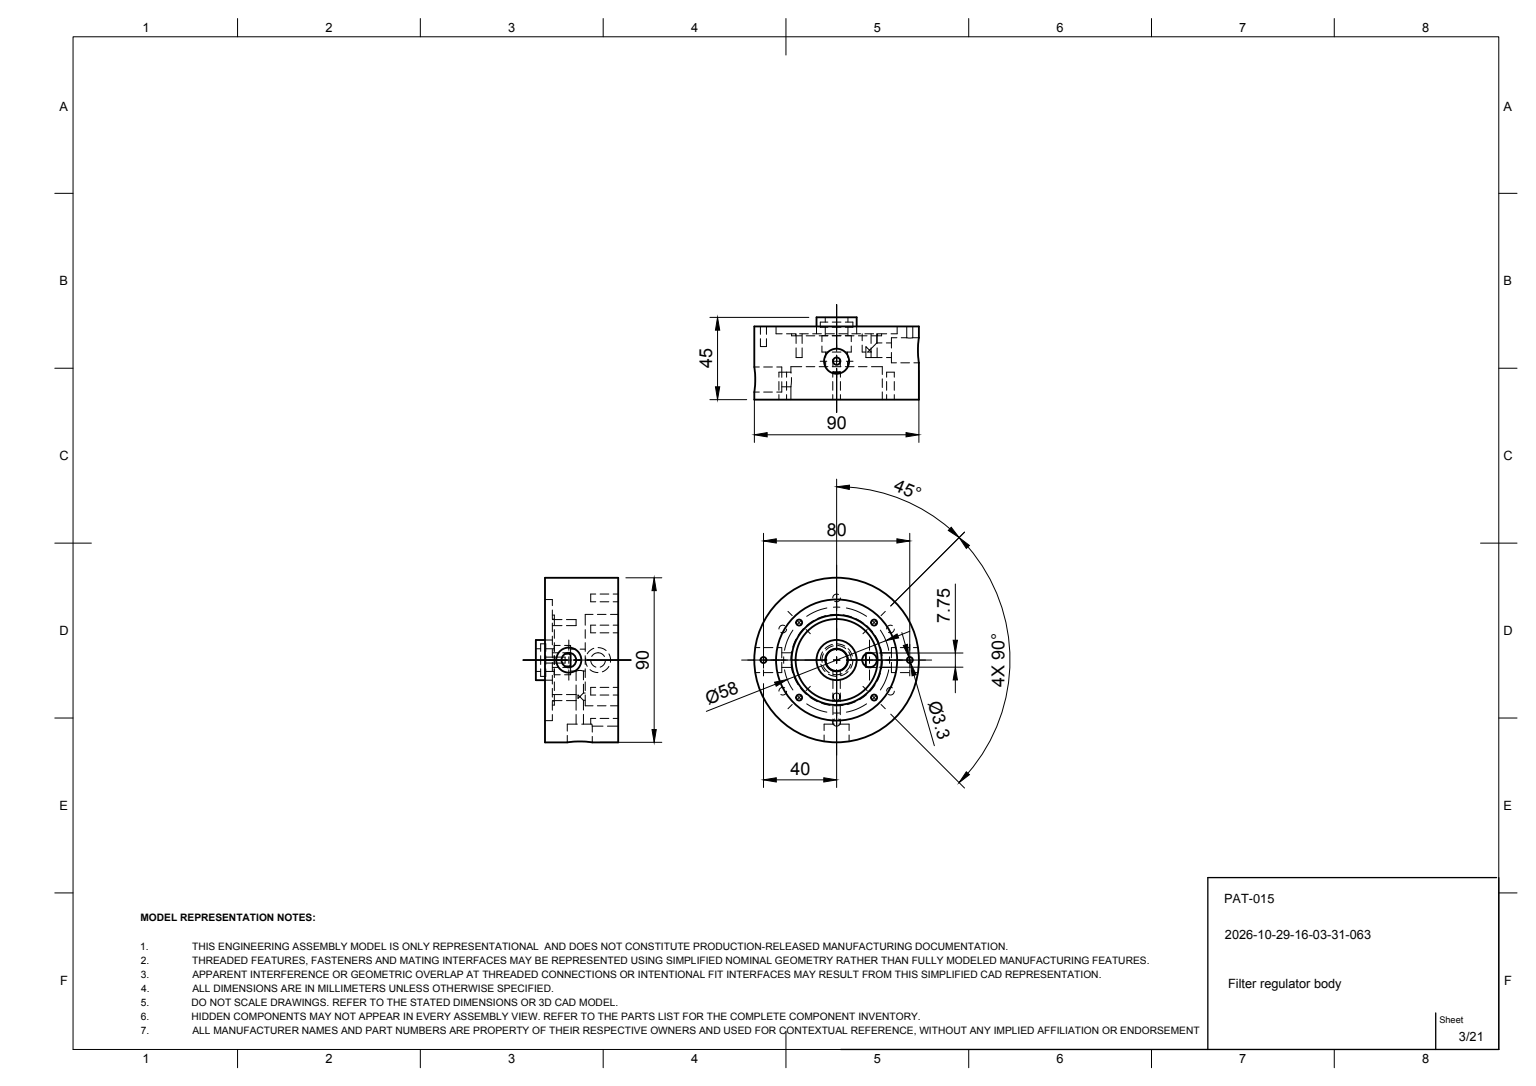
ISO-10303-21;
HEADER;
/* Generated by software containing ST-Developer
 * from STEP Tools, Inc. (www.steptools.com) 
 */

FILE_DESCRIPTION(
/* description */ ('PAT-015'),
/* implementation_level */ '2;1');

FILE_NAME(
/* name */ 'Filter regulator body.step',
/* time_stamp */ '2026-10-29T16:03:43-07:00',
/* author */ (''),
/* organization */ (''),
/* preprocessor_version */ 'ST-DEVELOPER v20.2',
/* originating_system */ 'Autodesk Translation Framework v15.17.0.0',
/* authorisation */ '');

FILE_SCHEMA (('AUTOMOTIVE_DESIGN { 1 0 10303 214 3 1 1 }'));
ENDSEC;

DATA;
#10=MECHANICAL_DESIGN_GEOMETRIC_PRESENTATION_REPRESENTATION('',(#230),#10266);
#184=SHAPE_REPRESENTATION_RELATIONSHIP('SRR','None',#10355,#207);
#207=ADVANCED_BREP_SHAPE_REPRESENTATION('',(#255),#10243);
#230=STYLED_ITEM('',(#10526),#255);
#255=MANIFOLD_SOLID_BREP('Body1',#4689);
#278=ELLIPSE('',#5037,0.282842712474619,0.2);
#279=ELLIPSE('',#5038,0.282842712474619,0.2);
#280=ELLIPSE('',#5040,0.282842712474619,0.2);
#281=ELLIPSE('',#5041,0.282842712474619,0.2);
#282=ELLIPSE('',#5043,0.282842712474619,0.2);
#283=ELLIPSE('',#5045,0.282842712474619,0.2);
#284=ELLIPSE('',#5060,0.565685424949238,0.4);
#285=ELLIPSE('',#5061,0.565685424949238,0.4);
#286=ELLIPSE('',#5063,0.565685424949238,0.4);
#287=ELLIPSE('',#5064,0.565685424949238,0.4);
#288=ELLIPSE('',#5067,0.565685424949238,0.4);
#289=ELLIPSE('',#5068,0.565685424949238,0.4);
#290=ELLIPSE('',#5069,0.565685424949238,0.4);
#291=ELLIPSE('',#5070,0.565685424949238,0.4);
#292=FACE_BOUND('',#868,.T.);
#293=FACE_BOUND('',#870,.T.);
#294=FACE_BOUND('',#871,.T.);
#295=FACE_BOUND('',#872,.T.);
#296=FACE_BOUND('',#873,.T.);
#297=FACE_BOUND('',#874,.T.);
#298=FACE_BOUND('',#888,.T.);
#299=FACE_BOUND('',#899,.T.);
#300=FACE_BOUND('',#909,.T.);
#301=FACE_BOUND('',#911,.T.);
#302=FACE_BOUND('',#914,.T.);
#303=FACE_BOUND('',#916,.T.);
#304=FACE_BOUND('',#921,.T.);
#305=FACE_BOUND('',#923,.T.);
#306=FACE_BOUND('',#925,.T.);
#307=FACE_BOUND('',#928,.T.);
#308=FACE_BOUND('',#930,.T.);
#309=FACE_BOUND('',#932,.T.);
#310=FACE_BOUND('',#933,.T.);
#311=FACE_BOUND('',#936,.T.);
#312=FACE_BOUND('',#937,.T.);
#313=FACE_BOUND('',#939,.T.);
#314=FACE_BOUND('',#940,.T.);
#315=FACE_BOUND('',#942,.T.);
#316=FACE_BOUND('',#943,.T.);
#317=FACE_BOUND('',#944,.T.);
#318=FACE_BOUND('',#945,.T.);
#319=FACE_BOUND('',#946,.T.);
#320=FACE_BOUND('',#947,.T.);
#321=FACE_BOUND('',#948,.T.);
#322=FACE_BOUND('',#950,.T.);
#323=FACE_BOUND('',#951,.T.);
#324=FACE_BOUND('',#952,.T.);
#420=PLANE('',#4977);
#421=PLANE('',#4981);
#422=PLANE('',#4985);
#423=PLANE('',#4989);
#424=PLANE('',#4993);
#425=PLANE('',#5000);
#426=PLANE('',#5001);
#427=PLANE('',#5003);
#428=PLANE('',#5011);
#429=PLANE('',#5015);
#430=PLANE('',#5019);
#431=PLANE('',#5023);
#432=PLANE('',#5027);
#433=PLANE('',#5028);
#434=PLANE('',#5032);
#435=PLANE('',#5034);
#436=PLANE('',#5052);
#437=PLANE('',#5053);
#438=PLANE('',#5055);
#439=PLANE('',#5057);
#440=PLANE('',#5071);
#441=PLANE('',#5078);
#442=PLANE('',#5082);
#443=PLANE('',#5084);
#444=PLANE('',#5093);
#445=PLANE('',#5095);
#446=PLANE('',#5101);
#447=PLANE('',#5105);
#448=PLANE('',#5108);
#449=PLANE('',#5112);
#450=PLANE('',#5113);
#571=FACE_OUTER_BOUND('',#854,.T.);
#572=FACE_OUTER_BOUND('',#855,.T.);
#573=FACE_OUTER_BOUND('',#856,.T.);
#574=FACE_OUTER_BOUND('',#857,.T.);
#575=FACE_OUTER_BOUND('',#858,.T.);
#576=FACE_OUTER_BOUND('',#859,.T.);
#577=FACE_OUTER_BOUND('',#860,.T.);
#578=FACE_OUTER_BOUND('',#861,.T.);
#579=FACE_OUTER_BOUND('',#862,.T.);
#580=FACE_OUTER_BOUND('',#863,.T.);
#581=FACE_OUTER_BOUND('',#864,.T.);
#582=FACE_OUTER_BOUND('',#865,.T.);
#583=FACE_OUTER_BOUND('',#866,.T.);
#584=FACE_OUTER_BOUND('',#867,.T.);
#585=FACE_OUTER_BOUND('',#869,.T.);
#586=FACE_OUTER_BOUND('',#875,.T.);
#587=FACE_OUTER_BOUND('',#876,.T.);
#588=FACE_OUTER_BOUND('',#877,.T.);
#589=FACE_OUTER_BOUND('',#878,.T.);
#590=FACE_OUTER_BOUND('',#879,.T.);
#591=FACE_OUTER_BOUND('',#880,.T.);
#592=FACE_OUTER_BOUND('',#881,.T.);
#593=FACE_OUTER_BOUND('',#882,.T.);
#594=FACE_OUTER_BOUND('',#883,.T.);
#595=FACE_OUTER_BOUND('',#884,.T.);
#596=FACE_OUTER_BOUND('',#885,.T.);
#597=FACE_OUTER_BOUND('',#886,.T.);
#598=FACE_OUTER_BOUND('',#887,.T.);
#599=FACE_OUTER_BOUND('',#889,.T.);
#600=FACE_OUTER_BOUND('',#890,.T.);
#601=FACE_OUTER_BOUND('',#891,.T.);
#602=FACE_OUTER_BOUND('',#892,.T.);
#603=FACE_OUTER_BOUND('',#893,.T.);
#604=FACE_OUTER_BOUND('',#894,.T.);
#605=FACE_OUTER_BOUND('',#895,.T.);
#606=FACE_OUTER_BOUND('',#896,.T.);
#607=FACE_OUTER_BOUND('',#897,.T.);
#608=FACE_OUTER_BOUND('',#898,.T.);
#609=FACE_OUTER_BOUND('',#900,.T.);
#610=FACE_OUTER_BOUND('',#901,.T.);
#611=FACE_OUTER_BOUND('',#902,.T.);
#612=FACE_OUTER_BOUND('',#903,.T.);
#613=FACE_OUTER_BOUND('',#904,.T.);
#614=FACE_OUTER_BOUND('',#905,.T.);
#615=FACE_OUTER_BOUND('',#906,.T.);
#616=FACE_OUTER_BOUND('',#907,.T.);
#617=FACE_OUTER_BOUND('',#908,.T.);
#618=FACE_OUTER_BOUND('',#910,.T.);
#619=FACE_OUTER_BOUND('',#912,.T.);
#620=FACE_OUTER_BOUND('',#913,.T.);
#621=FACE_OUTER_BOUND('',#915,.T.);
#622=FACE_OUTER_BOUND('',#917,.T.);
#623=FACE_OUTER_BOUND('',#918,.T.);
#624=FACE_OUTER_BOUND('',#919,.T.);
#625=FACE_OUTER_BOUND('',#920,.T.);
#626=FACE_OUTER_BOUND('',#922,.T.);
#627=FACE_OUTER_BOUND('',#924,.T.);
#628=FACE_OUTER_BOUND('',#926,.T.);
#629=FACE_OUTER_BOUND('',#927,.T.);
#630=FACE_OUTER_BOUND('',#929,.T.);
#631=FACE_OUTER_BOUND('',#931,.T.);
#632=FACE_OUTER_BOUND('',#934,.T.);
#633=FACE_OUTER_BOUND('',#935,.T.);
#634=FACE_OUTER_BOUND('',#938,.T.);
#635=FACE_OUTER_BOUND('',#941,.T.);
#636=FACE_OUTER_BOUND('',#949,.T.);
#854=EDGE_LOOP('',(#3101,#3102,#3103,#3104,#3105));
#855=EDGE_LOOP('',(#3106,#3107,#3108,#3109));
#856=EDGE_LOOP('',(#3110));
#857=EDGE_LOOP('',(#3111,#3112,#3113,#3114));
#858=EDGE_LOOP('',(#3115));
#859=EDGE_LOOP('',(#3116,#3117,#3118,#3119));
#860=EDGE_LOOP('',(#3120));
#861=EDGE_LOOP('',(#3121,#3122,#3123,#3124));
#862=EDGE_LOOP('',(#3125));
#863=EDGE_LOOP('',(#3126,#3127,#3128,#3129));
#864=EDGE_LOOP('',(#3130));
#865=EDGE_LOOP('',(#3131,#3132,#3133,#3134));
#866=EDGE_LOOP('',(#3135,#3136,#3137,#3138));
#867=EDGE_LOOP('',(#3139));
#868=EDGE_LOOP('',(#3140));
#869=EDGE_LOOP('',(#3141));
#870=EDGE_LOOP('',(#3142));
#871=EDGE_LOOP('',(#3143));
#872=EDGE_LOOP('',(#3144));
#873=EDGE_LOOP('',(#3145));
#874=EDGE_LOOP('',(#3146));
#875=EDGE_LOOP('',(#3147,#3148,#3149));
#876=EDGE_LOOP('',(#3150,#3151,#3152,#3153,#3154,#3155,#3156,#3157));
#877=EDGE_LOOP('',(#3158,#3159,#3160,#3161));
#878=EDGE_LOOP('',(#3162));
#879=EDGE_LOOP('',(#3163,#3164,#3165,#3166));
#880=EDGE_LOOP('',(#3167));
#881=EDGE_LOOP('',(#3168,#3169,#3170,#3171));
#882=EDGE_LOOP('',(#3172));
#883=EDGE_LOOP('',(#3173,#3174,#3175,#3176));
#884=EDGE_LOOP('',(#3177));
#885=EDGE_LOOP('',(#3178,#3179,#3180,#3181));
#886=EDGE_LOOP('',(#3182));
#887=EDGE_LOOP('',(#3183,#3184,#3185,#3186,#3187));
#888=EDGE_LOOP('',(#3188));
#889=EDGE_LOOP('',(#3189,#3190));
#890=EDGE_LOOP('',(#3191,#3192));
#891=EDGE_LOOP('',(#3193,#3194,#3195));
#892=EDGE_LOOP('',(#3196,#3197,#3198));
#893=EDGE_LOOP('',(#3199,#3200,#3201,#3202,#3203));
#894=EDGE_LOOP('',(#3204,#3205,#3206,#3207,#3208,#3209,#3210,#3211,#3212,
#3213,#3214,#3215,#3216,#3217));
#895=EDGE_LOOP('',(#3218,#3219,#3220,#3221,#3222,#3223));
#896=EDGE_LOOP('',(#3224,#3225,#3226,#3227,#3228));
#897=EDGE_LOOP('',(#3229,#3230,#3231,#3232,#3233));
#898=EDGE_LOOP('',(#3234));
#899=EDGE_LOOP('',(#3235));
#900=EDGE_LOOP('',(#3236,#3237));
#901=EDGE_LOOP('',(#3238,#3239));
#902=EDGE_LOOP('',(#3240,#3241));
#903=EDGE_LOOP('',(#3242,#3243,#3244));
#904=EDGE_LOOP('',(#3245,#3246,#3247));
#905=EDGE_LOOP('',(#3248,#3249,#3250,#3251,#3252,#3253,#3254,#3255,#3256,
#3257));
#906=EDGE_LOOP('',(#3258,#3259,#3260,#3261,#3262));
#907=EDGE_LOOP('',(#3263,#3264,#3265,#3266,#3267,#3268,#3269,#3270,#3271,
#3272,#3273,#3274,#3275,#3276,#3277));
#908=EDGE_LOOP('',(#3278,#3279,#3280,#3281,#3282,#3283));
#909=EDGE_LOOP('',(#3284,#3285));
#910=EDGE_LOOP('',(#3286));
#911=EDGE_LOOP('',(#3287));
#912=EDGE_LOOP('',(#3288,#3289,#3290,#3291));
#913=EDGE_LOOP('',(#3292));
#914=EDGE_LOOP('',(#3293));
#915=EDGE_LOOP('',(#3294));
#916=EDGE_LOOP('',(#3295));
#917=EDGE_LOOP('',(#3296,#3297,#3298,#3299));
#918=EDGE_LOOP('',(#3300,#3301,#3302,#3303));
#919=EDGE_LOOP('',(#3304,#3305,#3306,#3307));
#920=EDGE_LOOP('',(#3308));
#921=EDGE_LOOP('',(#3309));
#922=EDGE_LOOP('',(#3310));
#923=EDGE_LOOP('',(#3311));
#924=EDGE_LOOP('',(#3312,#3313,#3314,#3315));
#925=EDGE_LOOP('',(#3316));
#926=EDGE_LOOP('',(#3317,#3318,#3319,#3320));
#927=EDGE_LOOP('',(#3321));
#928=EDGE_LOOP('',(#3322));
#929=EDGE_LOOP('',(#3323,#3324,#3325,#3326));
#930=EDGE_LOOP('',(#3327,#3328));
#931=EDGE_LOOP('',(#3329));
#932=EDGE_LOOP('',(#3330));
#933=EDGE_LOOP('',(#3331));
#934=EDGE_LOOP('',(#3332,#3333,#3334,#3335));
#935=EDGE_LOOP('',(#3336));
#936=EDGE_LOOP('',(#3337));
#937=EDGE_LOOP('',(#3338));
#938=EDGE_LOOP('',(#3339,#3340,#3341,#3342,#3343,#3344,#3345,#3346,#3347));
#939=EDGE_LOOP('',(#3348));
#940=EDGE_LOOP('',(#3349,#3350));
#941=EDGE_LOOP('',(#3351));
#942=EDGE_LOOP('',(#3352));
#943=EDGE_LOOP('',(#3353));
#944=EDGE_LOOP('',(#3354));
#945=EDGE_LOOP('',(#3355));
#946=EDGE_LOOP('',(#3356));
#947=EDGE_LOOP('',(#3357));
#948=EDGE_LOOP('',(#3358));
#949=EDGE_LOOP('',(#3359));
#950=EDGE_LOOP('',(#3360));
#951=EDGE_LOOP('',(#3361));
#952=EDGE_LOOP('',(#3362));
#1265=B_SPLINE_CURVE_WITH_KNOTS('',3,(#7016,#7017,#7018,#7019,#7020,#7021,
#7022,#7023,#7024,#7025),.UNSPECIFIED.,.F.,.F.,(4,2,2,2,4),(0.,0.0624222198205065,
0.124844439641013,0.187259170559066,0.249673901477119),.UNSPECIFIED.);
#1266=B_SPLINE_CURVE_WITH_KNOTS('',3,(#7026,#7027,#7028,#7029,#7030,#7031,
#7032,#7033,#7034,#7035,#7036,#7037,#7038,#7039,#7040,#7041,#7042,#7043,
#7044,#7045,#7046,#7047,#7048,#7049,#7050,#7051),.UNSPECIFIED.,.F.,.F.,
(4,2,2,2,2,2,2,2,2,2,2,2,4),(0.249673901477119,0.312088632395172,0.374503363313225,
0.436925583133731,0.499347802954238,0.561770022774744,0.624192242595251,
0.686606973513304,0.749021704431357,0.811436435349409,0.873851166267462,
0.936273386087969,0.998695605908476),.UNSPECIFIED.);
#1267=B_SPLINE_CURVE_WITH_KNOTS('',3,(#7114,#7115,#7116,#7117,#7118,#7119,
#7120,#7121,#7122,#7123,#7124,#7125,#7126,#7127),.UNSPECIFIED.,.F.,.F.,
(4,2,2,2,2,2,4),(0.737404739505917,0.796636749554485,0.876284832373894,
0.955932915193303,1.03558099801271,1.11522908083212,1.17446109088069),
 .UNSPECIFIED.);
#1268=B_SPLINE_CURVE_WITH_KNOTS('',3,(#7201,#7202,#7203,#7204,#7205,#7206,
#7207,#7208,#7209,#7210,#7211,#7212,#7213,#7214,#7215,#7216,#7217,#7218,
#7219,#7220,#7221,#7222,#7223,#7224,#7225,#7226,#7227,#7228,#7229,#7230,
#7231,#7232,#7233,#7234),.UNSPECIFIED.,.T.,.F.,(4,2,2,2,2,2,2,2,2,2,2,2,
2,2,2,2,4),(0.,0.0759876362447374,0.151975272489475,0.227927665609886,0.303880058730296,
0.379832451850707,0.455784844971118,0.531772481215856,0.607760117460593,
0.68374775370533,0.759735389950068,0.835687783070479,0.911640176190889,
0.9875925693113,1.06354496243171,1.13953259867645,1.21552023492119),
 .UNSPECIFIED.);
#1269=B_SPLINE_CURVE_WITH_KNOTS('',3,(#7237,#7238,#7239,#7240,#7241,#7242,
#7243,#7244,#7245,#7246,#7247,#7248,#7249,#7250,#7251,#7252,#7253,#7254,
#7255,#7256,#7257,#7258,#7259,#7260,#7261,#7262,#7263,#7264,#7265,#7266,
#7267,#7268,#7269,#7270),.UNSPECIFIED.,.T.,.F.,(4,2,2,2,2,2,2,2,2,2,2,2,
2,2,2,2,4),(0.,0.258464867281583,0.516929734563166,0.775389819140497,1.03384990371783,
1.29230998829516,1.55077007287249,1.80923494015407,2.06769980743566,2.32616467471724,
2.58462954199882,2.84308962657615,3.10154971115348,3.36000979573081,3.61846988030814,
3.87693474758973,4.13539961487131),.UNSPECIFIED.);
#1270=B_SPLINE_CURVE_WITH_KNOTS('',3,(#7275,#7276,#7277,#7278,#7279,#7280,
#7281,#7282,#7283,#7284),.UNSPECIFIED.,.F.,.F.,(4,2,2,2,4),(0.,0.150955476673376,
0.301910953346751,0.452863012665493,0.603815071984235),.UNSPECIFIED.);
#1271=B_SPLINE_CURVE_WITH_KNOTS('',3,(#7285,#7286,#7287,#7288,#7289,#7290,
#7291,#7292,#7293,#7294,#7295,#7296,#7297,#7298,#7299,#7300,#7301,#7302,
#7303,#7304,#7305,#7306,#7307,#7308,#7309,#7310),.UNSPECIFIED.,.F.,.F.,
(4,2,2,2,2,2,2,2,2,2,2,2,4),(0.603815071984235,0.754767131302978,0.90571919062172,
1.0566746672951,1.20763014396847,1.35858562064185,1.50954109731522,1.66049315663396,
1.81144521595271,1.96239727527145,2.11334933459019,2.26430481126357,2.41526028793694),
 .UNSPECIFIED.);
#1272=B_SPLINE_CURVE_WITH_KNOTS('',3,(#7320,#7321,#7322,#7323,#7324,#7325,
#7326,#7327,#7328,#7329,#7330,#7331,#7332,#7333,#7334,#7335,#7336,#7337,
#7338,#7339,#7340,#7341,#7342,#7343,#7344,#7345),.UNSPECIFIED.,.F.,.F.,
(4,2,2,2,2,2,2,2,2,2,2,2,4),(0.,0.258464867281583,0.516929734563165,0.775389819140496,
1.03384990371783,1.29230998829516,1.55077007287249,1.80923494015407,2.06769980743565,
2.32616467471724,2.58462954199882,2.84308962657615,3.10154971115348),
 .UNSPECIFIED.);
#1273=B_SPLINE_CURVE_WITH_KNOTS('',3,(#7346,#7347,#7348,#7349,#7350,#7351,
#7352,#7353,#7354,#7355),.UNSPECIFIED.,.F.,.F.,(4,2,2,2,4),(3.10154971115348,
3.36000979573081,3.61846988030814,3.87693474758973,4.13539961487131),
 .UNSPECIFIED.);
#1274=B_SPLINE_CURVE_WITH_KNOTS('',3,(#7404,#7405,#7406,#7407,#7408,#7409,
#7410,#7411,#7412,#7413),.UNSPECIFIED.,.F.,.F.,(4,2,2,2,4),(0.,0.258464867281583,
0.516929734563165,0.775389819140497,1.03384990371783),.UNSPECIFIED.);
#1275=B_SPLINE_CURVE_WITH_KNOTS('',3,(#7415,#7416,#7417,#7418,#7419,#7420,
#7421,#7422,#7423,#7424),.UNSPECIFIED.,.F.,.F.,(4,2,2,2,4),(3.10154971115348,
3.36000979573081,3.61846988030815,3.87693474758973,4.13539961487131),
 .UNSPECIFIED.);
#1276=B_SPLINE_CURVE_WITH_KNOTS('',3,(#7425,#7426,#7427,#7428,#7429,#7430,
#7431,#7432,#7433,#7434,#7435,#7436,#7437,#7438,#7439,#7440,#7441,#7442),
 .UNSPECIFIED.,.F.,.F.,(4,2,2,2,2,2,2,2,4),(1.03384990371783,1.29230998829516,
1.55077007287249,1.80923494015407,2.06769980743566,2.32616467471724,2.58462954199882,
2.84308962657615,3.10154971115348),.UNSPECIFIED.);
#1323=LINE('',#7014,#1603);
#1324=LINE('',#7056,#1604);
#1325=LINE('',#7063,#1605);
#1326=LINE('',#7070,#1606);
#1327=LINE('',#7077,#1607);
#1328=LINE('',#7084,#1608);
#1329=LINE('',#7091,#1609);
#1330=LINE('',#7097,#1610);
#1331=LINE('',#7106,#1611);
#1332=LINE('',#7112,#1612);
#1333=LINE('',#7128,#1613);
#1334=LINE('',#7130,#1614);
#1335=LINE('',#7136,#1615);
#1336=LINE('',#7143,#1616);
#1337=LINE('',#7150,#1617);
#1338=LINE('',#7157,#1618);
#1339=LINE('',#7164,#1619);
#1340=LINE('',#7176,#1620);
#1341=LINE('',#7181,#1621);
#1342=LINE('',#7194,#1622);
#1343=LINE('',#7198,#1623);
#1344=LINE('',#7200,#1624);
#1345=LINE('',#7271,#1625);
#1346=LINE('',#7312,#1626);
#1347=LINE('',#7318,#1627);
#1348=LINE('',#7360,#1628);
#1349=LINE('',#7365,#1629);
#1350=LINE('',#7370,#1630);
#1351=LINE('',#7384,#1631);
#1352=LINE('',#7388,#1632);
#1353=LINE('',#7390,#1633);
#1354=LINE('',#7400,#1634);
#1355=LINE('',#7444,#1635);
#1356=LINE('',#7451,#1636);
#1357=LINE('',#7462,#1637);
#1358=LINE('',#7465,#1638);
#1359=LINE('',#7471,#1639);
#1360=LINE('',#7481,#1640);
#1361=LINE('',#7485,#1641);
#1362=LINE('',#7492,#1642);
#1363=LINE('',#7498,#1643);
#1364=LINE('',#7503,#1644);
#1365=LINE('',#7505,#1645);
#1603=VECTOR('',#5564,0.165);
#1604=VECTOR('',#5569,0.165);
#1605=VECTOR('',#5578,0.165);
#1606=VECTOR('',#5587,0.165);
#1607=VECTOR('',#5596,0.165);
#1608=VECTOR('',#5605,0.165);
#1609=VECTOR('',#5614,2.24);
#1610=VECTOR('',#5621,2.46);
#1611=VECTOR('',#5632,1.);
#1612=VECTOR('',#5639,1.);
#1613=VECTOR('',#5640,1.);
#1614=VECTOR('',#5641,0.21);
#1615=VECTOR('',#5648,0.21);
#1616=VECTOR('',#5657,0.21);
#1617=VECTOR('',#5666,0.21);
#1618=VECTOR('',#5675,0.21);
#1619=VECTOR('',#5684,0.21);
#1620=VECTOR('',#5699,1.);
#1621=VECTOR('',#5704,1.);
#1622=VECTOR('',#5723,0.2);
#1623=VECTOR('',#5730,0.2);
#1624=VECTOR('',#5731,0.2);
#1625=VECTOR('',#5734,0.685);
#1626=VECTOR('',#5737,0.4);
#1627=VECTOR('',#5744,0.685);
#1628=VECTOR('',#5749,1.);
#1629=VECTOR('',#5754,1.);
#1630=VECTOR('',#5759,1.);
#1631=VECTOR('',#5778,0.4);
#1632=VECTOR('',#5783,1.);
#1633=VECTOR('',#5784,1.);
#1634=VECTOR('',#5799,0.4);
#1635=VECTOR('',#5802,0.685);
#1636=VECTOR('',#5811,0.89);
#1637=VECTOR('',#5826,0.6185);
#1638=VECTOR('',#5829,0.6185);
#1639=VECTOR('',#5836,1.1);
#1640=VECTOR('',#5849,0.6);
#1641=VECTOR('',#5854,0.8);
#1642=VECTOR('',#5863,2.5);
#1643=VECTOR('',#5872,3.31);
#1644=VECTOR('',#5879,4.5);
#1645=VECTOR('',#5880,4.5);
#1883=CIRCLE('',#4973,0.165);
#1884=CIRCLE('',#4975,0.165);
#1885=CIRCLE('',#4976,0.165);
#1886=CIRCLE('',#4979,0.165);
#1887=CIRCLE('',#4980,0.165);
#1888=CIRCLE('',#4983,0.165);
#1889=CIRCLE('',#4984,0.165);
#1890=CIRCLE('',#4987,0.165);
#1891=CIRCLE('',#4988,0.165);
#1892=CIRCLE('',#4991,0.165);
#1893=CIRCLE('',#4992,0.165);
#1894=CIRCLE('',#4995,2.24);
#1895=CIRCLE('',#4996,2.24);
#1896=CIRCLE('',#4998,2.46);
#1897=CIRCLE('',#4999,2.46);
#1898=CIRCLE('',#5002,3.31);
#1899=CIRCLE('',#5004,0.21);
#1900=CIRCLE('',#5005,0.21);
#1901=CIRCLE('',#5007,0.21);
#1902=CIRCLE('',#5009,0.21);
#1903=CIRCLE('',#5010,0.21);
#1904=CIRCLE('',#5013,0.21);
#1905=CIRCLE('',#5014,0.21);
#1906=CIRCLE('',#5017,0.21);
#1907=CIRCLE('',#5018,0.21);
#1908=CIRCLE('',#5021,0.21);
#1909=CIRCLE('',#5022,0.21);
#1910=CIRCLE('',#5025,0.21);
#1911=CIRCLE('',#5026,0.21);
#1912=CIRCLE('',#5029,0.685);
#1913=CIRCLE('',#5030,0.685);
#1914=CIRCLE('',#5031,0.2);
#1915=CIRCLE('',#5033,0.2);
#1916=CIRCLE('',#5035,0.2);
#1917=CIRCLE('',#5044,0.2);
#1918=CIRCLE('',#5049,0.4);
#1919=CIRCLE('',#5051,0.685);
#1920=CIRCLE('',#5054,0.4);
#1921=CIRCLE('',#5056,0.4);
#1922=CIRCLE('',#5058,0.4);
#1923=CIRCLE('',#5066,0.4);
#1924=CIRCLE('',#5072,0.4);
#1925=CIRCLE('',#5073,0.4);
#1926=CIRCLE('',#5075,0.4);
#1927=CIRCLE('',#5077,0.685);
#1928=CIRCLE('',#5080,0.89);
#1929=CIRCLE('',#5081,0.89);
#1930=CIRCLE('',#5083,0.6185);
#1931=CIRCLE('',#5085,0.6185);
#1932=CIRCLE('',#5087,0.6185);
#1933=CIRCLE('',#5089,0.6185);
#1934=CIRCLE('',#5091,1.1);
#1935=CIRCLE('',#5092,1.1);
#1936=CIRCLE('',#5094,0.8);
#1937=CIRCLE('',#5097,0.6);
#1938=CIRCLE('',#5098,0.6);
#1939=CIRCLE('',#5100,0.8);
#1940=CIRCLE('',#5103,2.5);
#1941=CIRCLE('',#5104,2.5);
#1942=CIRCLE('',#5107,3.31);
#1943=CIRCLE('',#5110,4.5);
#1944=CIRCLE('',#5111,4.5);
#2114=VERTEX_POINT('',#7011);
#2115=VERTEX_POINT('',#7013);
#2116=VERTEX_POINT('',#7015);
#2117=VERTEX_POINT('',#7053);
#2118=VERTEX_POINT('',#7055);
#2119=VERTEX_POINT('',#7060);
#2120=VERTEX_POINT('',#7062);
#2121=VERTEX_POINT('',#7067);
#2122=VERTEX_POINT('',#7069);
#2123=VERTEX_POINT('',#7074);
#2124=VERTEX_POINT('',#7076);
#2125=VERTEX_POINT('',#7081);
#2126=VERTEX_POINT('',#7083);
#2127=VERTEX_POINT('',#7088);
#2128=VERTEX_POINT('',#7090);
#2129=VERTEX_POINT('',#7094);
#2130=VERTEX_POINT('',#7096);
#2131=VERTEX_POINT('',#7101);
#2132=VERTEX_POINT('',#7104);
#2133=VERTEX_POINT('',#7105);
#2134=VERTEX_POINT('',#7107);
#2135=VERTEX_POINT('',#7111);
#2136=VERTEX_POINT('',#7113);
#2137=VERTEX_POINT('',#7129);
#2138=VERTEX_POINT('',#7133);
#2139=VERTEX_POINT('',#7135);
#2140=VERTEX_POINT('',#7140);
#2141=VERTEX_POINT('',#7142);
#2142=VERTEX_POINT('',#7147);
#2143=VERTEX_POINT('',#7149);
#2144=VERTEX_POINT('',#7154);
#2145=VERTEX_POINT('',#7156);
#2146=VERTEX_POINT('',#7161);
#2147=VERTEX_POINT('',#7163);
#2148=VERTEX_POINT('',#7168);
#2149=VERTEX_POINT('',#7171);
#2150=VERTEX_POINT('',#7174);
#2151=VERTEX_POINT('',#7175);
#2152=VERTEX_POINT('',#7179);
#2153=VERTEX_POINT('',#7180);
#2154=VERTEX_POINT('',#7184);
#2155=VERTEX_POINT('',#7188);
#2156=VERTEX_POINT('',#7193);
#2157=VERTEX_POINT('',#7199);
#2158=VERTEX_POINT('',#7236);
#2159=VERTEX_POINT('',#7273);
#2160=VERTEX_POINT('',#7274);
#2161=VERTEX_POINT('',#7311);
#2162=VERTEX_POINT('',#7315);
#2163=VERTEX_POINT('',#7317);
#2164=VERTEX_POINT('',#7319);
#2165=VERTEX_POINT('',#7358);
#2166=VERTEX_POINT('',#7359);
#2167=VERTEX_POINT('',#7363);
#2168=VERTEX_POINT('',#7364);
#2169=VERTEX_POINT('',#7368);
#2170=VERTEX_POINT('',#7369);
#2171=VERTEX_POINT('',#7373);
#2172=VERTEX_POINT('',#7377);
#2173=VERTEX_POINT('',#7381);
#2174=VERTEX_POINT('',#7383);
#2175=VERTEX_POINT('',#7386);
#2176=VERTEX_POINT('',#7389);
#2177=VERTEX_POINT('',#7394);
#2178=VERTEX_POINT('',#7398);
#2179=VERTEX_POINT('',#7402);
#2180=VERTEX_POINT('',#7403);
#2181=VERTEX_POINT('',#7414);
#2182=VERTEX_POINT('',#7443);
#2183=VERTEX_POINT('',#7448);
#2184=VERTEX_POINT('',#7450);
#2185=VERTEX_POINT('',#7454);
#2186=VERTEX_POINT('',#7457);
#2187=VERTEX_POINT('',#7460);
#2188=VERTEX_POINT('',#7464);
#2189=VERTEX_POINT('',#7468);
#2190=VERTEX_POINT('',#7470);
#2191=VERTEX_POINT('',#7474);
#2192=VERTEX_POINT('',#7478);
#2193=VERTEX_POINT('',#7480);
#2194=VERTEX_POINT('',#7484);
#2195=VERTEX_POINT('',#7489);
#2196=VERTEX_POINT('',#7491);
#2197=VERTEX_POINT('',#7496);
#2198=VERTEX_POINT('',#7501);
#2199=VERTEX_POINT('',#7504);
#2506=EDGE_CURVE('',#2114,#2114,#1883,.T.);
#2507=EDGE_CURVE('',#2114,#2115,#1323,.T.);
#2508=EDGE_CURVE('',#2116,#2115,#1265,.T.);
#2509=EDGE_CURVE('',#2115,#2116,#1266,.T.);
#2510=EDGE_CURVE('',#2117,#2117,#1884,.T.);
#2511=EDGE_CURVE('',#2117,#2118,#1324,.T.);
#2512=EDGE_CURVE('',#2118,#2118,#1885,.T.);
#2513=EDGE_CURVE('',#2119,#2119,#1886,.T.);
#2514=EDGE_CURVE('',#2119,#2120,#1325,.T.);
#2515=EDGE_CURVE('',#2120,#2120,#1887,.T.);
#2516=EDGE_CURVE('',#2121,#2121,#1888,.T.);
#2517=EDGE_CURVE('',#2121,#2122,#1326,.T.);
#2518=EDGE_CURVE('',#2122,#2122,#1889,.T.);
#2519=EDGE_CURVE('',#2123,#2123,#1890,.T.);
#2520=EDGE_CURVE('',#2123,#2124,#1327,.T.);
#2521=EDGE_CURVE('',#2124,#2124,#1891,.T.);
#2522=EDGE_CURVE('',#2125,#2125,#1892,.T.);
#2523=EDGE_CURVE('',#2125,#2126,#1328,.T.);
#2524=EDGE_CURVE('',#2126,#2126,#1893,.T.);
#2525=EDGE_CURVE('',#2127,#2127,#1894,.T.);
#2526=EDGE_CURVE('',#2127,#2128,#1329,.T.);
#2527=EDGE_CURVE('',#2128,#2128,#1895,.T.);
#2528=EDGE_CURVE('',#2129,#2129,#1896,.T.);
#2529=EDGE_CURVE('',#2129,#2130,#1330,.T.);
#2530=EDGE_CURVE('',#2130,#2130,#1897,.T.);
#2531=EDGE_CURVE('',#2131,#2131,#1898,.T.);
#2532=EDGE_CURVE('',#2132,#2133,#1331,.T.);
#2533=EDGE_CURVE('',#2132,#2134,#1899,.T.);
#2534=EDGE_CURVE('',#2134,#2133,#1900,.T.);
#2535=EDGE_CURVE('',#2135,#2132,#1332,.T.);
#2536=EDGE_CURVE('',#2136,#2135,#1267,.T.);
#2537=EDGE_CURVE('',#2133,#2136,#1333,.T.);
#2538=EDGE_CURVE('',#2134,#2137,#1334,.T.);
#2539=EDGE_CURVE('',#2137,#2137,#1901,.T.);
#2540=EDGE_CURVE('',#2138,#2138,#1902,.T.);
#2541=EDGE_CURVE('',#2138,#2139,#1335,.T.);
#2542=EDGE_CURVE('',#2139,#2139,#1903,.T.);
#2543=EDGE_CURVE('',#2140,#2140,#1904,.T.);
#2544=EDGE_CURVE('',#2140,#2141,#1336,.T.);
#2545=EDGE_CURVE('',#2141,#2141,#1905,.T.);
#2546=EDGE_CURVE('',#2142,#2142,#1906,.T.);
#2547=EDGE_CURVE('',#2142,#2143,#1337,.T.);
#2548=EDGE_CURVE('',#2143,#2143,#1907,.T.);
#2549=EDGE_CURVE('',#2144,#2144,#1908,.T.);
#2550=EDGE_CURVE('',#2144,#2145,#1338,.T.);
#2551=EDGE_CURVE('',#2145,#2145,#1909,.T.);
#2552=EDGE_CURVE('',#2146,#2146,#1910,.T.);
#2553=EDGE_CURVE('',#2146,#2147,#1339,.T.);
#2554=EDGE_CURVE('',#2147,#2147,#1911,.T.);
#2555=EDGE_CURVE('',#2148,#2136,#1912,.T.);
#2556=EDGE_CURVE('',#2135,#2148,#1913,.T.);
#2557=EDGE_CURVE('',#2149,#2149,#1914,.T.);
#2558=EDGE_CURVE('',#2150,#2151,#1340,.T.);
#2559=EDGE_CURVE('',#2150,#2151,#1915,.T.);
#2560=EDGE_CURVE('',#2152,#2153,#1341,.T.);
#2561=EDGE_CURVE('',#2152,#2153,#1916,.T.);
#2562=EDGE_CURVE('',#2154,#2150,#278,.T.);
#2563=EDGE_CURVE('',#2151,#2154,#279,.T.);
#2564=EDGE_CURVE('',#2155,#2152,#280,.T.);
#2565=EDGE_CURVE('',#2153,#2155,#281,.T.);
#2566=EDGE_CURVE('',#2154,#2155,#282,.T.);
#2567=EDGE_CURVE('',#2154,#2156,#1342,.T.);
#2568=EDGE_CURVE('',#2156,#2156,#1917,.T.);
#2569=EDGE_CURVE('',#2155,#2154,#283,.T.);
#2570=EDGE_CURVE('',#2149,#2154,#1343,.T.);
#2571=EDGE_CURVE('',#2154,#2157,#1344,.T.);
#2572=EDGE_CURVE('',#2157,#2157,#1268,.T.);
#2573=EDGE_CURVE('',#2158,#2158,#1269,.T.);
#2574=EDGE_CURVE('',#2158,#2148,#1345,.T.);
#2575=EDGE_CURVE('',#2159,#2160,#1270,.T.);
#2576=EDGE_CURVE('',#2160,#2159,#1271,.T.);
#2577=EDGE_CURVE('',#2160,#2161,#1346,.T.);
#2578=EDGE_CURVE('',#2161,#2161,#1918,.T.);
#2579=EDGE_CURVE('',#2162,#2162,#1919,.T.);
#2580=EDGE_CURVE('',#2162,#2163,#1347,.T.);
#2581=EDGE_CURVE('',#2164,#2163,#1272,.T.);
#2582=EDGE_CURVE('',#2163,#2164,#1273,.T.);
#2583=EDGE_CURVE('',#2165,#2166,#1348,.T.);
#2584=EDGE_CURVE('',#2166,#2165,#1920,.T.);
#2585=EDGE_CURVE('',#2167,#2168,#1349,.T.);
#2586=EDGE_CURVE('',#2168,#2167,#1921,.T.);
#2587=EDGE_CURVE('',#2169,#2170,#1350,.T.);
#2588=EDGE_CURVE('',#2170,#2169,#1922,.T.);
#2589=EDGE_CURVE('',#2166,#2171,#284,.T.);
#2590=EDGE_CURVE('',#2171,#2165,#285,.T.);
#2591=EDGE_CURVE('',#2168,#2172,#286,.T.);
#2592=EDGE_CURVE('',#2172,#2167,#287,.T.);
#2593=EDGE_CURVE('',#2173,#2173,#1923,.T.);
#2594=EDGE_CURVE('',#2173,#2174,#1351,.T.);
#2595=EDGE_CURVE('',#2171,#2174,#288,.T.);
#2596=EDGE_CURVE('',#2175,#2171,#289,.T.);
#2597=EDGE_CURVE('',#2170,#2175,#1352,.T.);
#2598=EDGE_CURVE('',#2176,#2169,#1353,.T.);
#2599=EDGE_CURVE('',#2172,#2176,#290,.T.);
#2600=EDGE_CURVE('',#2174,#2172,#291,.T.);
#2601=EDGE_CURVE('',#2177,#2175,#1924,.T.);
#2602=EDGE_CURVE('',#2176,#2177,#1925,.T.);
#2603=EDGE_CURVE('',#2178,#2178,#1926,.T.);
#2604=EDGE_CURVE('',#2178,#2177,#1354,.T.);
#2605=EDGE_CURVE('',#2179,#2180,#1274,.T.);
#2606=EDGE_CURVE('',#2181,#2179,#1275,.T.);
#2607=EDGE_CURVE('',#2180,#2181,#1276,.T.);
#2608=EDGE_CURVE('',#2180,#2182,#1355,.T.);
#2609=EDGE_CURVE('',#2182,#2182,#1927,.T.);
#2610=EDGE_CURVE('',#2183,#2183,#1928,.T.);
#2611=EDGE_CURVE('',#2183,#2184,#1356,.T.);
#2612=EDGE_CURVE('',#2184,#2184,#1929,.T.);
#2613=EDGE_CURVE('',#2185,#2185,#1930,.T.);
#2614=EDGE_CURVE('',#2186,#2186,#1931,.T.);
#2615=EDGE_CURVE('',#2187,#2187,#1932,.T.);
#2616=EDGE_CURVE('',#2187,#2186,#1357,.T.);
#2617=EDGE_CURVE('',#2185,#2188,#1358,.T.);
#2618=EDGE_CURVE('',#2188,#2188,#1933,.T.);
#2619=EDGE_CURVE('',#2189,#2189,#1934,.T.);
#2620=EDGE_CURVE('',#2189,#2190,#1359,.T.);
#2621=EDGE_CURVE('',#2190,#2190,#1935,.T.);
#2622=EDGE_CURVE('',#2191,#2191,#1936,.T.);
#2623=EDGE_CURVE('',#2192,#2192,#1937,.T.);
#2624=EDGE_CURVE('',#2192,#2193,#1360,.T.);
#2625=EDGE_CURVE('',#2193,#2193,#1938,.T.);
#2626=EDGE_CURVE('',#2191,#2194,#1361,.T.);
#2627=EDGE_CURVE('',#2194,#2194,#1939,.T.);
#2628=EDGE_CURVE('',#2195,#2195,#1940,.T.);
#2629=EDGE_CURVE('',#2195,#2196,#1362,.T.);
#2630=EDGE_CURVE('',#2196,#2196,#1941,.T.);
#2631=EDGE_CURVE('',#2197,#2197,#1942,.T.);
#2632=EDGE_CURVE('',#2197,#2131,#1363,.T.);
#2633=EDGE_CURVE('',#2198,#2198,#1943,.T.);
#2634=EDGE_CURVE('',#2198,#2180,#1364,.T.);
#2635=EDGE_CURVE('',#2181,#2199,#1365,.T.);
#2636=EDGE_CURVE('',#2199,#2199,#1944,.T.);
#3101=ORIENTED_EDGE('',*,*,#2506,.F.);
#3102=ORIENTED_EDGE('',*,*,#2507,.T.);
#3103=ORIENTED_EDGE('',*,*,#2508,.F.);
#3104=ORIENTED_EDGE('',*,*,#2509,.F.);
#3105=ORIENTED_EDGE('',*,*,#2507,.F.);
#3106=ORIENTED_EDGE('',*,*,#2510,.F.);
#3107=ORIENTED_EDGE('',*,*,#2511,.T.);
#3108=ORIENTED_EDGE('',*,*,#2512,.T.);
#3109=ORIENTED_EDGE('',*,*,#2511,.F.);
#3110=ORIENTED_EDGE('',*,*,#2512,.F.);
#3111=ORIENTED_EDGE('',*,*,#2513,.F.);
#3112=ORIENTED_EDGE('',*,*,#2514,.T.);
#3113=ORIENTED_EDGE('',*,*,#2515,.T.);
#3114=ORIENTED_EDGE('',*,*,#2514,.F.);
#3115=ORIENTED_EDGE('',*,*,#2515,.F.);
#3116=ORIENTED_EDGE('',*,*,#2516,.F.);
#3117=ORIENTED_EDGE('',*,*,#2517,.T.);
#3118=ORIENTED_EDGE('',*,*,#2518,.T.);
#3119=ORIENTED_EDGE('',*,*,#2517,.F.);
#3120=ORIENTED_EDGE('',*,*,#2518,.F.);
#3121=ORIENTED_EDGE('',*,*,#2519,.F.);
#3122=ORIENTED_EDGE('',*,*,#2520,.T.);
#3123=ORIENTED_EDGE('',*,*,#2521,.T.);
#3124=ORIENTED_EDGE('',*,*,#2520,.F.);
#3125=ORIENTED_EDGE('',*,*,#2521,.F.);
#3126=ORIENTED_EDGE('',*,*,#2522,.F.);
#3127=ORIENTED_EDGE('',*,*,#2523,.T.);
#3128=ORIENTED_EDGE('',*,*,#2524,.T.);
#3129=ORIENTED_EDGE('',*,*,#2523,.F.);
#3130=ORIENTED_EDGE('',*,*,#2524,.F.);
#3131=ORIENTED_EDGE('',*,*,#2525,.F.);
#3132=ORIENTED_EDGE('',*,*,#2526,.T.);
#3133=ORIENTED_EDGE('',*,*,#2527,.T.);
#3134=ORIENTED_EDGE('',*,*,#2526,.F.);
#3135=ORIENTED_EDGE('',*,*,#2528,.F.);
#3136=ORIENTED_EDGE('',*,*,#2529,.T.);
#3137=ORIENTED_EDGE('',*,*,#2530,.T.);
#3138=ORIENTED_EDGE('',*,*,#2529,.F.);
#3139=ORIENTED_EDGE('',*,*,#2530,.F.);
#3140=ORIENTED_EDGE('',*,*,#2527,.F.);
#3141=ORIENTED_EDGE('',*,*,#2531,.F.);
#3142=ORIENTED_EDGE('',*,*,#2528,.T.);
#3143=ORIENTED_EDGE('',*,*,#2522,.T.);
#3144=ORIENTED_EDGE('',*,*,#2519,.T.);
#3145=ORIENTED_EDGE('',*,*,#2516,.T.);
#3146=ORIENTED_EDGE('',*,*,#2513,.T.);
#3147=ORIENTED_EDGE('',*,*,#2532,.F.);
#3148=ORIENTED_EDGE('',*,*,#2533,.T.);
#3149=ORIENTED_EDGE('',*,*,#2534,.T.);
#3150=ORIENTED_EDGE('',*,*,#2535,.F.);
#3151=ORIENTED_EDGE('',*,*,#2536,.F.);
#3152=ORIENTED_EDGE('',*,*,#2537,.F.);
#3153=ORIENTED_EDGE('',*,*,#2534,.F.);
#3154=ORIENTED_EDGE('',*,*,#2538,.T.);
#3155=ORIENTED_EDGE('',*,*,#2539,.F.);
#3156=ORIENTED_EDGE('',*,*,#2538,.F.);
#3157=ORIENTED_EDGE('',*,*,#2533,.F.);
#3158=ORIENTED_EDGE('',*,*,#2540,.F.);
#3159=ORIENTED_EDGE('',*,*,#2541,.T.);
#3160=ORIENTED_EDGE('',*,*,#2542,.F.);
#3161=ORIENTED_EDGE('',*,*,#2541,.F.);
#3162=ORIENTED_EDGE('',*,*,#2540,.T.);
#3163=ORIENTED_EDGE('',*,*,#2543,.F.);
#3164=ORIENTED_EDGE('',*,*,#2544,.T.);
#3165=ORIENTED_EDGE('',*,*,#2545,.F.);
#3166=ORIENTED_EDGE('',*,*,#2544,.F.);
#3167=ORIENTED_EDGE('',*,*,#2543,.T.);
#3168=ORIENTED_EDGE('',*,*,#2546,.F.);
#3169=ORIENTED_EDGE('',*,*,#2547,.T.);
#3170=ORIENTED_EDGE('',*,*,#2548,.F.);
#3171=ORIENTED_EDGE('',*,*,#2547,.F.);
#3172=ORIENTED_EDGE('',*,*,#2546,.T.);
#3173=ORIENTED_EDGE('',*,*,#2549,.F.);
#3174=ORIENTED_EDGE('',*,*,#2550,.T.);
#3175=ORIENTED_EDGE('',*,*,#2551,.F.);
#3176=ORIENTED_EDGE('',*,*,#2550,.F.);
#3177=ORIENTED_EDGE('',*,*,#2549,.T.);
#3178=ORIENTED_EDGE('',*,*,#2552,.F.);
#3179=ORIENTED_EDGE('',*,*,#2553,.T.);
#3180=ORIENTED_EDGE('',*,*,#2554,.F.);
#3181=ORIENTED_EDGE('',*,*,#2553,.F.);
#3182=ORIENTED_EDGE('',*,*,#2552,.T.);
#3183=ORIENTED_EDGE('',*,*,#2535,.T.);
#3184=ORIENTED_EDGE('',*,*,#2532,.T.);
#3185=ORIENTED_EDGE('',*,*,#2537,.T.);
#3186=ORIENTED_EDGE('',*,*,#2555,.F.);
#3187=ORIENTED_EDGE('',*,*,#2556,.F.);
#3188=ORIENTED_EDGE('',*,*,#2557,.T.);
#3189=ORIENTED_EDGE('',*,*,#2558,.F.);
#3190=ORIENTED_EDGE('',*,*,#2559,.T.);
#3191=ORIENTED_EDGE('',*,*,#2560,.F.);
#3192=ORIENTED_EDGE('',*,*,#2561,.T.);
#3193=ORIENTED_EDGE('',*,*,#2562,.F.);
#3194=ORIENTED_EDGE('',*,*,#2563,.F.);
#3195=ORIENTED_EDGE('',*,*,#2559,.F.);
#3196=ORIENTED_EDGE('',*,*,#2564,.F.);
#3197=ORIENTED_EDGE('',*,*,#2565,.F.);
#3198=ORIENTED_EDGE('',*,*,#2561,.F.);
#3199=ORIENTED_EDGE('',*,*,#2566,.F.);
#3200=ORIENTED_EDGE('',*,*,#2567,.T.);
#3201=ORIENTED_EDGE('',*,*,#2568,.F.);
#3202=ORIENTED_EDGE('',*,*,#2567,.F.);
#3203=ORIENTED_EDGE('',*,*,#2569,.F.);
#3204=ORIENTED_EDGE('',*,*,#2557,.F.);
#3205=ORIENTED_EDGE('',*,*,#2570,.T.);
#3206=ORIENTED_EDGE('',*,*,#2566,.T.);
#3207=ORIENTED_EDGE('',*,*,#2564,.T.);
#3208=ORIENTED_EDGE('',*,*,#2560,.T.);
#3209=ORIENTED_EDGE('',*,*,#2565,.T.);
#3210=ORIENTED_EDGE('',*,*,#2569,.T.);
#3211=ORIENTED_EDGE('',*,*,#2571,.T.);
#3212=ORIENTED_EDGE('',*,*,#2572,.F.);
#3213=ORIENTED_EDGE('',*,*,#2571,.F.);
#3214=ORIENTED_EDGE('',*,*,#2562,.T.);
#3215=ORIENTED_EDGE('',*,*,#2558,.T.);
#3216=ORIENTED_EDGE('',*,*,#2563,.T.);
#3217=ORIENTED_EDGE('',*,*,#2570,.F.);
#3218=ORIENTED_EDGE('',*,*,#2573,.F.);
#3219=ORIENTED_EDGE('',*,*,#2574,.T.);
#3220=ORIENTED_EDGE('',*,*,#2555,.T.);
#3221=ORIENTED_EDGE('',*,*,#2536,.T.);
#3222=ORIENTED_EDGE('',*,*,#2556,.T.);
#3223=ORIENTED_EDGE('',*,*,#2574,.F.);
#3224=ORIENTED_EDGE('',*,*,#2575,.F.);
#3225=ORIENTED_EDGE('',*,*,#2576,.F.);
#3226=ORIENTED_EDGE('',*,*,#2577,.T.);
#3227=ORIENTED_EDGE('',*,*,#2578,.F.);
#3228=ORIENTED_EDGE('',*,*,#2577,.F.);
#3229=ORIENTED_EDGE('',*,*,#2579,.F.);
#3230=ORIENTED_EDGE('',*,*,#2580,.T.);
#3231=ORIENTED_EDGE('',*,*,#2581,.F.);
#3232=ORIENTED_EDGE('',*,*,#2582,.F.);
#3233=ORIENTED_EDGE('',*,*,#2580,.F.);
#3234=ORIENTED_EDGE('',*,*,#2579,.T.);
#3235=ORIENTED_EDGE('',*,*,#2578,.T.);
#3236=ORIENTED_EDGE('',*,*,#2583,.F.);
#3237=ORIENTED_EDGE('',*,*,#2584,.F.);
#3238=ORIENTED_EDGE('',*,*,#2585,.F.);
#3239=ORIENTED_EDGE('',*,*,#2586,.F.);
#3240=ORIENTED_EDGE('',*,*,#2587,.F.);
#3241=ORIENTED_EDGE('',*,*,#2588,.F.);
#3242=ORIENTED_EDGE('',*,*,#2589,.F.);
#3243=ORIENTED_EDGE('',*,*,#2584,.T.);
#3244=ORIENTED_EDGE('',*,*,#2590,.F.);
#3245=ORIENTED_EDGE('',*,*,#2591,.F.);
#3246=ORIENTED_EDGE('',*,*,#2586,.T.);
#3247=ORIENTED_EDGE('',*,*,#2592,.F.);
#3248=ORIENTED_EDGE('',*,*,#2593,.F.);
#3249=ORIENTED_EDGE('',*,*,#2594,.T.);
#3250=ORIENTED_EDGE('',*,*,#2595,.F.);
#3251=ORIENTED_EDGE('',*,*,#2596,.F.);
#3252=ORIENTED_EDGE('',*,*,#2597,.F.);
#3253=ORIENTED_EDGE('',*,*,#2588,.T.);
#3254=ORIENTED_EDGE('',*,*,#2598,.F.);
#3255=ORIENTED_EDGE('',*,*,#2599,.F.);
#3256=ORIENTED_EDGE('',*,*,#2600,.F.);
#3257=ORIENTED_EDGE('',*,*,#2594,.F.);
#3258=ORIENTED_EDGE('',*,*,#2598,.T.);
#3259=ORIENTED_EDGE('',*,*,#2587,.T.);
#3260=ORIENTED_EDGE('',*,*,#2597,.T.);
#3261=ORIENTED_EDGE('',*,*,#2601,.F.);
#3262=ORIENTED_EDGE('',*,*,#2602,.F.);
#3263=ORIENTED_EDGE('',*,*,#2603,.F.);
#3264=ORIENTED_EDGE('',*,*,#2604,.T.);
#3265=ORIENTED_EDGE('',*,*,#2601,.T.);
#3266=ORIENTED_EDGE('',*,*,#2596,.T.);
#3267=ORIENTED_EDGE('',*,*,#2590,.T.);
#3268=ORIENTED_EDGE('',*,*,#2583,.T.);
#3269=ORIENTED_EDGE('',*,*,#2589,.T.);
#3270=ORIENTED_EDGE('',*,*,#2595,.T.);
#3271=ORIENTED_EDGE('',*,*,#2600,.T.);
#3272=ORIENTED_EDGE('',*,*,#2592,.T.);
#3273=ORIENTED_EDGE('',*,*,#2585,.T.);
#3274=ORIENTED_EDGE('',*,*,#2591,.T.);
#3275=ORIENTED_EDGE('',*,*,#2599,.T.);
#3276=ORIENTED_EDGE('',*,*,#2602,.T.);
#3277=ORIENTED_EDGE('',*,*,#2604,.F.);
#3278=ORIENTED_EDGE('',*,*,#2605,.F.);
#3279=ORIENTED_EDGE('',*,*,#2606,.F.);
#3280=ORIENTED_EDGE('',*,*,#2607,.F.);
#3281=ORIENTED_EDGE('',*,*,#2608,.T.);
#3282=ORIENTED_EDGE('',*,*,#2609,.T.);
#3283=ORIENTED_EDGE('',*,*,#2608,.F.);
#3284=ORIENTED_EDGE('',*,*,#2508,.T.);
#3285=ORIENTED_EDGE('',*,*,#2509,.T.);
#3286=ORIENTED_EDGE('',*,*,#2609,.F.);
#3287=ORIENTED_EDGE('',*,*,#2603,.T.);
#3288=ORIENTED_EDGE('',*,*,#2610,.F.);
#3289=ORIENTED_EDGE('',*,*,#2611,.T.);
#3290=ORIENTED_EDGE('',*,*,#2612,.T.);
#3291=ORIENTED_EDGE('',*,*,#2611,.F.);
#3292=ORIENTED_EDGE('',*,*,#2612,.F.);
#3293=ORIENTED_EDGE('',*,*,#2613,.F.);
#3294=ORIENTED_EDGE('',*,*,#2610,.T.);
#3295=ORIENTED_EDGE('',*,*,#2614,.F.);
#3296=ORIENTED_EDGE('',*,*,#2615,.F.);
#3297=ORIENTED_EDGE('',*,*,#2616,.T.);
#3298=ORIENTED_EDGE('',*,*,#2614,.T.);
#3299=ORIENTED_EDGE('',*,*,#2616,.F.);
#3300=ORIENTED_EDGE('',*,*,#2613,.T.);
#3301=ORIENTED_EDGE('',*,*,#2617,.T.);
#3302=ORIENTED_EDGE('',*,*,#2618,.F.);
#3303=ORIENTED_EDGE('',*,*,#2617,.F.);
#3304=ORIENTED_EDGE('',*,*,#2619,.F.);
#3305=ORIENTED_EDGE('',*,*,#2620,.T.);
#3306=ORIENTED_EDGE('',*,*,#2621,.T.);
#3307=ORIENTED_EDGE('',*,*,#2620,.F.);
#3308=ORIENTED_EDGE('',*,*,#2622,.F.);
#3309=ORIENTED_EDGE('',*,*,#2618,.T.);
#3310=ORIENTED_EDGE('',*,*,#2621,.F.);
#3311=ORIENTED_EDGE('',*,*,#2615,.T.);
#3312=ORIENTED_EDGE('',*,*,#2623,.F.);
#3313=ORIENTED_EDGE('',*,*,#2624,.T.);
#3314=ORIENTED_EDGE('',*,*,#2625,.F.);
#3315=ORIENTED_EDGE('',*,*,#2624,.F.);
#3316=ORIENTED_EDGE('',*,*,#2572,.T.);
#3317=ORIENTED_EDGE('',*,*,#2622,.T.);
#3318=ORIENTED_EDGE('',*,*,#2626,.T.);
#3319=ORIENTED_EDGE('',*,*,#2627,.T.);
#3320=ORIENTED_EDGE('',*,*,#2626,.F.);
#3321=ORIENTED_EDGE('',*,*,#2627,.F.);
#3322=ORIENTED_EDGE('',*,*,#2623,.T.);
#3323=ORIENTED_EDGE('',*,*,#2628,.F.);
#3324=ORIENTED_EDGE('',*,*,#2629,.T.);
#3325=ORIENTED_EDGE('',*,*,#2630,.F.);
#3326=ORIENTED_EDGE('',*,*,#2629,.F.);
#3327=ORIENTED_EDGE('',*,*,#2575,.T.);
#3328=ORIENTED_EDGE('',*,*,#2576,.T.);
#3329=ORIENTED_EDGE('',*,*,#2628,.T.);
#3330=ORIENTED_EDGE('',*,*,#2568,.T.);
#3331=ORIENTED_EDGE('',*,*,#2625,.T.);
#3332=ORIENTED_EDGE('',*,*,#2631,.F.);
#3333=ORIENTED_EDGE('',*,*,#2632,.T.);
#3334=ORIENTED_EDGE('',*,*,#2531,.T.);
#3335=ORIENTED_EDGE('',*,*,#2632,.F.);
#3336=ORIENTED_EDGE('',*,*,#2525,.T.);
#3337=ORIENTED_EDGE('',*,*,#2593,.T.);
#3338=ORIENTED_EDGE('',*,*,#2619,.T.);
#3339=ORIENTED_EDGE('',*,*,#2633,.F.);
#3340=ORIENTED_EDGE('',*,*,#2634,.T.);
#3341=ORIENTED_EDGE('',*,*,#2607,.T.);
#3342=ORIENTED_EDGE('',*,*,#2635,.T.);
#3343=ORIENTED_EDGE('',*,*,#2636,.T.);
#3344=ORIENTED_EDGE('',*,*,#2635,.F.);
#3345=ORIENTED_EDGE('',*,*,#2606,.T.);
#3346=ORIENTED_EDGE('',*,*,#2605,.T.);
#3347=ORIENTED_EDGE('',*,*,#2634,.F.);
#3348=ORIENTED_EDGE('',*,*,#2573,.T.);
#3349=ORIENTED_EDGE('',*,*,#2581,.T.);
#3350=ORIENTED_EDGE('',*,*,#2582,.T.);
#3351=ORIENTED_EDGE('',*,*,#2633,.T.);
#3352=ORIENTED_EDGE('',*,*,#2630,.T.);
#3353=ORIENTED_EDGE('',*,*,#2554,.T.);
#3354=ORIENTED_EDGE('',*,*,#2551,.T.);
#3355=ORIENTED_EDGE('',*,*,#2548,.T.);
#3356=ORIENTED_EDGE('',*,*,#2545,.T.);
#3357=ORIENTED_EDGE('',*,*,#2542,.T.);
#3358=ORIENTED_EDGE('',*,*,#2539,.T.);
#3359=ORIENTED_EDGE('',*,*,#2636,.F.);
#3360=ORIENTED_EDGE('',*,*,#2506,.T.);
#3361=ORIENTED_EDGE('',*,*,#2510,.T.);
#3362=ORIENTED_EDGE('',*,*,#2631,.T.);
#4291=CYLINDRICAL_SURFACE('',#4972,0.165);
#4292=CYLINDRICAL_SURFACE('',#4974,0.165);
#4293=CYLINDRICAL_SURFACE('',#4978,0.165);
#4294=CYLINDRICAL_SURFACE('',#4982,0.165);
#4295=CYLINDRICAL_SURFACE('',#4986,0.165);
#4296=CYLINDRICAL_SURFACE('',#4990,0.165);
#4297=CYLINDRICAL_SURFACE('',#4994,2.24);
#4298=CYLINDRICAL_SURFACE('',#4997,2.46);
#4299=CYLINDRICAL_SURFACE('',#5006,0.21);
#4300=CYLINDRICAL_SURFACE('',#5008,0.21);
#4301=CYLINDRICAL_SURFACE('',#5012,0.21);
#4302=CYLINDRICAL_SURFACE('',#5016,0.21);
#4303=CYLINDRICAL_SURFACE('',#5020,0.21);
#4304=CYLINDRICAL_SURFACE('',#5024,0.21);
#4305=CYLINDRICAL_SURFACE('',#5036,0.2);
#4306=CYLINDRICAL_SURFACE('',#5039,0.2);
#4307=CYLINDRICAL_SURFACE('',#5042,0.2);
#4308=CYLINDRICAL_SURFACE('',#5046,0.2);
#4309=CYLINDRICAL_SURFACE('',#5047,0.685);
#4310=CYLINDRICAL_SURFACE('',#5048,0.4);
#4311=CYLINDRICAL_SURFACE('',#5050,0.685);
#4312=CYLINDRICAL_SURFACE('',#5059,0.4);
#4313=CYLINDRICAL_SURFACE('',#5062,0.4);
#4314=CYLINDRICAL_SURFACE('',#5065,0.4);
#4315=CYLINDRICAL_SURFACE('',#5074,0.4);
#4316=CYLINDRICAL_SURFACE('',#5076,0.685);
#4317=CYLINDRICAL_SURFACE('',#5079,0.89);
#4318=CYLINDRICAL_SURFACE('',#5086,0.6185);
#4319=CYLINDRICAL_SURFACE('',#5088,0.6185);
#4320=CYLINDRICAL_SURFACE('',#5090,1.1);
#4321=CYLINDRICAL_SURFACE('',#5096,0.6);
#4322=CYLINDRICAL_SURFACE('',#5099,0.8);
#4323=CYLINDRICAL_SURFACE('',#5102,2.5);
#4324=CYLINDRICAL_SURFACE('',#5106,3.31);
#4325=CYLINDRICAL_SURFACE('',#5109,4.5);
#4406=ADVANCED_FACE('',(#571),#4291,.F.);
#4407=ADVANCED_FACE('',(#572),#4292,.F.);
#4408=ADVANCED_FACE('',(#573),#420,.F.);
#4409=ADVANCED_FACE('',(#574),#4293,.F.);
#4410=ADVANCED_FACE('',(#575),#421,.F.);
#4411=ADVANCED_FACE('',(#576),#4294,.F.);
#4412=ADVANCED_FACE('',(#577),#422,.F.);
#4413=ADVANCED_FACE('',(#578),#4295,.F.);
#4414=ADVANCED_FACE('',(#579),#423,.F.);
#4415=ADVANCED_FACE('',(#580),#4296,.F.);
#4416=ADVANCED_FACE('',(#581),#424,.F.);
#4417=ADVANCED_FACE('',(#582),#4297,.T.);
#4418=ADVANCED_FACE('',(#583),#4298,.F.);
#4419=ADVANCED_FACE('',(#584,#292),#425,.F.);
#4420=ADVANCED_FACE('',(#585,#293,#294,#295,#296,#297),#426,.F.);
#4421=ADVANCED_FACE('',(#586),#427,.T.);
#4422=ADVANCED_FACE('',(#587),#4299,.F.);
#4423=ADVANCED_FACE('',(#588),#4300,.F.);
#4424=ADVANCED_FACE('',(#589),#428,.T.);
#4425=ADVANCED_FACE('',(#590),#4301,.F.);
#4426=ADVANCED_FACE('',(#591),#429,.T.);
#4427=ADVANCED_FACE('',(#592),#4302,.F.);
#4428=ADVANCED_FACE('',(#593),#430,.T.);
#4429=ADVANCED_FACE('',(#594),#4303,.F.);
#4430=ADVANCED_FACE('',(#595),#431,.T.);
#4431=ADVANCED_FACE('',(#596),#4304,.F.);
#4432=ADVANCED_FACE('',(#597),#432,.T.);
#4433=ADVANCED_FACE('',(#598,#298),#433,.F.);
#4434=ADVANCED_FACE('',(#599),#434,.T.);
#4435=ADVANCED_FACE('',(#600),#435,.T.);
#4436=ADVANCED_FACE('',(#601),#4305,.F.);
#4437=ADVANCED_FACE('',(#602),#4306,.F.);
#4438=ADVANCED_FACE('',(#603),#4307,.F.);
#4439=ADVANCED_FACE('',(#604),#4308,.F.);
#4440=ADVANCED_FACE('',(#605),#4309,.F.);
#4441=ADVANCED_FACE('',(#606),#4310,.F.);
#4442=ADVANCED_FACE('',(#607),#4311,.F.);
#4443=ADVANCED_FACE('',(#608,#299),#436,.T.);
#4444=ADVANCED_FACE('',(#609),#437,.F.);
#4445=ADVANCED_FACE('',(#610),#438,.F.);
#4446=ADVANCED_FACE('',(#611),#439,.F.);
#4447=ADVANCED_FACE('',(#612),#4312,.F.);
#4448=ADVANCED_FACE('',(#613),#4313,.F.);
#4449=ADVANCED_FACE('',(#614),#4314,.F.);
#4450=ADVANCED_FACE('',(#615),#440,.F.);
#4451=ADVANCED_FACE('',(#616),#4315,.F.);
#4452=ADVANCED_FACE('',(#617,#300),#4316,.F.);
#4453=ADVANCED_FACE('',(#618,#301),#441,.F.);
#4454=ADVANCED_FACE('',(#619),#4317,.F.);
#4455=ADVANCED_FACE('',(#620,#302),#442,.F.);
#4456=ADVANCED_FACE('',(#621,#303),#443,.T.);
#4457=ADVANCED_FACE('',(#622),#4318,.F.);
#4458=ADVANCED_FACE('',(#623),#4319,.F.);
#4459=ADVANCED_FACE('',(#624),#4320,.T.);
#4460=ADVANCED_FACE('',(#625,#304),#444,.T.);
#4461=ADVANCED_FACE('',(#626,#305),#445,.F.);
#4462=ADVANCED_FACE('',(#627,#306),#4321,.F.);
#4463=ADVANCED_FACE('',(#628),#4322,.F.);
#4464=ADVANCED_FACE('',(#629,#307),#446,.F.);
#4465=ADVANCED_FACE('',(#630,#308),#4323,.F.);
#4466=ADVANCED_FACE('',(#631,#309,#310),#447,.T.);
#4467=ADVANCED_FACE('',(#632),#4324,.F.);
#4468=ADVANCED_FACE('',(#633,#311,#312),#448,.F.);
#4469=ADVANCED_FACE('',(#634,#313,#314),#4325,.T.);
#4470=ADVANCED_FACE('',(#635,#315,#316,#317,#318,#319,#320,#321),#449,.T.);
#4471=ADVANCED_FACE('',(#636,#322,#323,#324),#450,.F.);
#4689=CLOSED_SHELL('',(#4406,#4407,#4408,#4409,#4410,#4411,#4412,#4413,
#4414,#4415,#4416,#4417,#4418,#4419,#4420,#4421,#4422,#4423,#4424,#4425,
#4426,#4427,#4428,#4429,#4430,#4431,#4432,#4433,#4434,#4435,#4436,#4437,
#4438,#4439,#4440,#4441,#4442,#4443,#4444,#4445,#4446,#4447,#4448,#4449,
#4450,#4451,#4452,#4453,#4454,#4455,#4456,#4457,#4458,#4459,#4460,#4461,
#4462,#4463,#4464,#4465,#4466,#4467,#4468,#4469,#4470,#4471));
#4971=AXIS2_PLACEMENT_3D('',#7009,#5558,#5559);
#4972=AXIS2_PLACEMENT_3D('',#7010,#5560,#5561);
#4973=AXIS2_PLACEMENT_3D('',#7012,#5562,#5563);
#4974=AXIS2_PLACEMENT_3D('',#7052,#5565,#5566);
#4975=AXIS2_PLACEMENT_3D('',#7054,#5567,#5568);
#4976=AXIS2_PLACEMENT_3D('',#7057,#5570,#5571);
#4977=AXIS2_PLACEMENT_3D('',#7058,#5572,#5573);
#4978=AXIS2_PLACEMENT_3D('',#7059,#5574,#5575);
#4979=AXIS2_PLACEMENT_3D('',#7061,#5576,#5577);
#4980=AXIS2_PLACEMENT_3D('',#7064,#5579,#5580);
#4981=AXIS2_PLACEMENT_3D('',#7065,#5581,#5582);
#4982=AXIS2_PLACEMENT_3D('',#7066,#5583,#5584);
#4983=AXIS2_PLACEMENT_3D('',#7068,#5585,#5586);
#4984=AXIS2_PLACEMENT_3D('',#7071,#5588,#5589);
#4985=AXIS2_PLACEMENT_3D('',#7072,#5590,#5591);
#4986=AXIS2_PLACEMENT_3D('',#7073,#5592,#5593);
#4987=AXIS2_PLACEMENT_3D('',#7075,#5594,#5595);
#4988=AXIS2_PLACEMENT_3D('',#7078,#5597,#5598);
#4989=AXIS2_PLACEMENT_3D('',#7079,#5599,#5600);
#4990=AXIS2_PLACEMENT_3D('',#7080,#5601,#5602);
#4991=AXIS2_PLACEMENT_3D('',#7082,#5603,#5604);
#4992=AXIS2_PLACEMENT_3D('',#7085,#5606,#5607);
#4993=AXIS2_PLACEMENT_3D('',#7086,#5608,#5609);
#4994=AXIS2_PLACEMENT_3D('',#7087,#5610,#5611);
#4995=AXIS2_PLACEMENT_3D('',#7089,#5612,#5613);
#4996=AXIS2_PLACEMENT_3D('',#7092,#5615,#5616);
#4997=AXIS2_PLACEMENT_3D('',#7093,#5617,#5618);
#4998=AXIS2_PLACEMENT_3D('',#7095,#5619,#5620);
#4999=AXIS2_PLACEMENT_3D('',#7098,#5622,#5623);
#5000=AXIS2_PLACEMENT_3D('',#7099,#5624,#5625);
#5001=AXIS2_PLACEMENT_3D('',#7100,#5626,#5627);
#5002=AXIS2_PLACEMENT_3D('',#7102,#5628,#5629);
#5003=AXIS2_PLACEMENT_3D('',#7103,#5630,#5631);
#5004=AXIS2_PLACEMENT_3D('',#7108,#5633,#5634);
#5005=AXIS2_PLACEMENT_3D('',#7109,#5635,#5636);
#5006=AXIS2_PLACEMENT_3D('',#7110,#5637,#5638);
#5007=AXIS2_PLACEMENT_3D('',#7131,#5642,#5643);
#5008=AXIS2_PLACEMENT_3D('',#7132,#5644,#5645);
#5009=AXIS2_PLACEMENT_3D('',#7134,#5646,#5647);
#5010=AXIS2_PLACEMENT_3D('',#7137,#5649,#5650);
#5011=AXIS2_PLACEMENT_3D('',#7138,#5651,#5652);
#5012=AXIS2_PLACEMENT_3D('',#7139,#5653,#5654);
#5013=AXIS2_PLACEMENT_3D('',#7141,#5655,#5656);
#5014=AXIS2_PLACEMENT_3D('',#7144,#5658,#5659);
#5015=AXIS2_PLACEMENT_3D('',#7145,#5660,#5661);
#5016=AXIS2_PLACEMENT_3D('',#7146,#5662,#5663);
#5017=AXIS2_PLACEMENT_3D('',#7148,#5664,#5665);
#5018=AXIS2_PLACEMENT_3D('',#7151,#5667,#5668);
#5019=AXIS2_PLACEMENT_3D('',#7152,#5669,#5670);
#5020=AXIS2_PLACEMENT_3D('',#7153,#5671,#5672);
#5021=AXIS2_PLACEMENT_3D('',#7155,#5673,#5674);
#5022=AXIS2_PLACEMENT_3D('',#7158,#5676,#5677);
#5023=AXIS2_PLACEMENT_3D('',#7159,#5678,#5679);
#5024=AXIS2_PLACEMENT_3D('',#7160,#5680,#5681);
#5025=AXIS2_PLACEMENT_3D('',#7162,#5682,#5683);
#5026=AXIS2_PLACEMENT_3D('',#7165,#5685,#5686);
#5027=AXIS2_PLACEMENT_3D('',#7166,#5687,#5688);
#5028=AXIS2_PLACEMENT_3D('',#7167,#5689,#5690);
#5029=AXIS2_PLACEMENT_3D('',#7169,#5691,#5692);
#5030=AXIS2_PLACEMENT_3D('',#7170,#5693,#5694);
#5031=AXIS2_PLACEMENT_3D('',#7172,#5695,#5696);
#5032=AXIS2_PLACEMENT_3D('',#7173,#5697,#5698);
#5033=AXIS2_PLACEMENT_3D('',#7177,#5700,#5701);
#5034=AXIS2_PLACEMENT_3D('',#7178,#5702,#5703);
#5035=AXIS2_PLACEMENT_3D('',#7182,#5705,#5706);
#5036=AXIS2_PLACEMENT_3D('',#7183,#5707,#5708);
#5037=AXIS2_PLACEMENT_3D('',#7185,#5709,#5710);
#5038=AXIS2_PLACEMENT_3D('',#7186,#5711,#5712);
#5039=AXIS2_PLACEMENT_3D('',#7187,#5713,#5714);
#5040=AXIS2_PLACEMENT_3D('',#7189,#5715,#5716);
#5041=AXIS2_PLACEMENT_3D('',#7190,#5717,#5718);
#5042=AXIS2_PLACEMENT_3D('',#7191,#5719,#5720);
#5043=AXIS2_PLACEMENT_3D('',#7192,#5721,#5722);
#5044=AXIS2_PLACEMENT_3D('',#7195,#5724,#5725);
#5045=AXIS2_PLACEMENT_3D('',#7196,#5726,#5727);
#5046=AXIS2_PLACEMENT_3D('',#7197,#5728,#5729);
#5047=AXIS2_PLACEMENT_3D('',#7235,#5732,#5733);
#5048=AXIS2_PLACEMENT_3D('',#7272,#5735,#5736);
#5049=AXIS2_PLACEMENT_3D('',#7313,#5738,#5739);
#5050=AXIS2_PLACEMENT_3D('',#7314,#5740,#5741);
#5051=AXIS2_PLACEMENT_3D('',#7316,#5742,#5743);
#5052=AXIS2_PLACEMENT_3D('',#7356,#5745,#5746);
#5053=AXIS2_PLACEMENT_3D('',#7357,#5747,#5748);
#5054=AXIS2_PLACEMENT_3D('',#7361,#5750,#5751);
#5055=AXIS2_PLACEMENT_3D('',#7362,#5752,#5753);
#5056=AXIS2_PLACEMENT_3D('',#7366,#5755,#5756);
#5057=AXIS2_PLACEMENT_3D('',#7367,#5757,#5758);
#5058=AXIS2_PLACEMENT_3D('',#7371,#5760,#5761);
#5059=AXIS2_PLACEMENT_3D('',#7372,#5762,#5763);
#5060=AXIS2_PLACEMENT_3D('',#7374,#5764,#5765);
#5061=AXIS2_PLACEMENT_3D('',#7375,#5766,#5767);
#5062=AXIS2_PLACEMENT_3D('',#7376,#5768,#5769);
#5063=AXIS2_PLACEMENT_3D('',#7378,#5770,#5771);
#5064=AXIS2_PLACEMENT_3D('',#7379,#5772,#5773);
#5065=AXIS2_PLACEMENT_3D('',#7380,#5774,#5775);
#5066=AXIS2_PLACEMENT_3D('',#7382,#5776,#5777);
#5067=AXIS2_PLACEMENT_3D('',#7385,#5779,#5780);
#5068=AXIS2_PLACEMENT_3D('',#7387,#5781,#5782);
#5069=AXIS2_PLACEMENT_3D('',#7391,#5785,#5786);
#5070=AXIS2_PLACEMENT_3D('',#7392,#5787,#5788);
#5071=AXIS2_PLACEMENT_3D('',#7393,#5789,#5790);
#5072=AXIS2_PLACEMENT_3D('',#7395,#5791,#5792);
#5073=AXIS2_PLACEMENT_3D('',#7396,#5793,#5794);
#5074=AXIS2_PLACEMENT_3D('',#7397,#5795,#5796);
#5075=AXIS2_PLACEMENT_3D('',#7399,#5797,#5798);
#5076=AXIS2_PLACEMENT_3D('',#7401,#5800,#5801);
#5077=AXIS2_PLACEMENT_3D('',#7445,#5803,#5804);
#5078=AXIS2_PLACEMENT_3D('',#7446,#5805,#5806);
#5079=AXIS2_PLACEMENT_3D('',#7447,#5807,#5808);
#5080=AXIS2_PLACEMENT_3D('',#7449,#5809,#5810);
#5081=AXIS2_PLACEMENT_3D('',#7452,#5812,#5813);
#5082=AXIS2_PLACEMENT_3D('',#7453,#5814,#5815);
#5083=AXIS2_PLACEMENT_3D('',#7455,#5816,#5817);
#5084=AXIS2_PLACEMENT_3D('',#7456,#5818,#5819);
#5085=AXIS2_PLACEMENT_3D('',#7458,#5820,#5821);
#5086=AXIS2_PLACEMENT_3D('',#7459,#5822,#5823);
#5087=AXIS2_PLACEMENT_3D('',#7461,#5824,#5825);
#5088=AXIS2_PLACEMENT_3D('',#7463,#5827,#5828);
#5089=AXIS2_PLACEMENT_3D('',#7466,#5830,#5831);
#5090=AXIS2_PLACEMENT_3D('',#7467,#5832,#5833);
#5091=AXIS2_PLACEMENT_3D('',#7469,#5834,#5835);
#5092=AXIS2_PLACEMENT_3D('',#7472,#5837,#5838);
#5093=AXIS2_PLACEMENT_3D('',#7473,#5839,#5840);
#5094=AXIS2_PLACEMENT_3D('',#7475,#5841,#5842);
#5095=AXIS2_PLACEMENT_3D('',#7476,#5843,#5844);
#5096=AXIS2_PLACEMENT_3D('',#7477,#5845,#5846);
#5097=AXIS2_PLACEMENT_3D('',#7479,#5847,#5848);
#5098=AXIS2_PLACEMENT_3D('',#7482,#5850,#5851);
#5099=AXIS2_PLACEMENT_3D('',#7483,#5852,#5853);
#5100=AXIS2_PLACEMENT_3D('',#7486,#5855,#5856);
#5101=AXIS2_PLACEMENT_3D('',#7487,#5857,#5858);
#5102=AXIS2_PLACEMENT_3D('',#7488,#5859,#5860);
#5103=AXIS2_PLACEMENT_3D('',#7490,#5861,#5862);
#5104=AXIS2_PLACEMENT_3D('',#7493,#5864,#5865);
#5105=AXIS2_PLACEMENT_3D('',#7494,#5866,#5867);
#5106=AXIS2_PLACEMENT_3D('',#7495,#5868,#5869);
#5107=AXIS2_PLACEMENT_3D('',#7497,#5870,#5871);
#5108=AXIS2_PLACEMENT_3D('',#7499,#5873,#5874);
#5109=AXIS2_PLACEMENT_3D('',#7500,#5875,#5876);
#5110=AXIS2_PLACEMENT_3D('',#7502,#5877,#5878);
#5111=AXIS2_PLACEMENT_3D('',#7506,#5881,#5882);
#5112=AXIS2_PLACEMENT_3D('',#7507,#5883,#5884);
#5113=AXIS2_PLACEMENT_3D('',#7508,#5885,#5886);
#5558=DIRECTION('axis',(0.,0.,1.));
#5559=DIRECTION('refdir',(1.,0.,0.));
#5560=DIRECTION('center_axis',(0.,0.,1.));
#5561=DIRECTION('ref_axis',(1.,0.,0.));
#5562=DIRECTION('center_axis',(0.,0.,1.));
#5563=DIRECTION('ref_axis',(1.,0.,0.));
#5564=DIRECTION('',(0.,0.,1.));
#5565=DIRECTION('center_axis',(0.,0.,1.));
#5566=DIRECTION('ref_axis',(1.,0.,0.));
#5567=DIRECTION('center_axis',(0.,0.,1.));
#5568=DIRECTION('ref_axis',(1.,0.,0.));
#5569=DIRECTION('',(0.,0.,1.));
#5570=DIRECTION('center_axis',(0.,0.,1.));
#5571=DIRECTION('ref_axis',(1.,0.,0.));
#5572=DIRECTION('center_axis',(0.,0.,1.));
#5573=DIRECTION('ref_axis',(1.,0.,0.));
#5574=DIRECTION('center_axis',(0.,0.,1.));
#5575=DIRECTION('ref_axis',(1.,0.,0.));
#5576=DIRECTION('center_axis',(0.,0.,1.));
#5577=DIRECTION('ref_axis',(1.,0.,0.));
#5578=DIRECTION('',(0.,0.,1.));
#5579=DIRECTION('center_axis',(0.,0.,1.));
#5580=DIRECTION('ref_axis',(1.,0.,0.));
#5581=DIRECTION('center_axis',(0.,0.,1.));
#5582=DIRECTION('ref_axis',(1.,0.,0.));
#5583=DIRECTION('center_axis',(0.,0.,1.));
#5584=DIRECTION('ref_axis',(1.,0.,0.));
#5585=DIRECTION('center_axis',(0.,0.,1.));
#5586=DIRECTION('ref_axis',(1.,0.,0.));
#5587=DIRECTION('',(0.,0.,1.));
#5588=DIRECTION('center_axis',(0.,0.,1.));
#5589=DIRECTION('ref_axis',(1.,0.,0.));
#5590=DIRECTION('center_axis',(0.,0.,1.));
#5591=DIRECTION('ref_axis',(1.,0.,0.));
#5592=DIRECTION('center_axis',(0.,0.,1.));
#5593=DIRECTION('ref_axis',(1.,0.,0.));
#5594=DIRECTION('center_axis',(0.,0.,1.));
#5595=DIRECTION('ref_axis',(1.,0.,0.));
#5596=DIRECTION('',(0.,0.,1.));
#5597=DIRECTION('center_axis',(0.,0.,1.));
#5598=DIRECTION('ref_axis',(1.,0.,0.));
#5599=DIRECTION('center_axis',(0.,0.,1.));
#5600=DIRECTION('ref_axis',(1.,0.,0.));
#5601=DIRECTION('center_axis',(0.,0.,1.));
#5602=DIRECTION('ref_axis',(1.,0.,0.));
#5603=DIRECTION('center_axis',(0.,0.,1.));
#5604=DIRECTION('ref_axis',(1.,0.,0.));
#5605=DIRECTION('',(0.,0.,1.));
#5606=DIRECTION('center_axis',(0.,0.,1.));
#5607=DIRECTION('ref_axis',(1.,0.,0.));
#5608=DIRECTION('center_axis',(0.,0.,1.));
#5609=DIRECTION('ref_axis',(1.,0.,0.));
#5610=DIRECTION('center_axis',(0.,0.,1.));
#5611=DIRECTION('ref_axis',(1.,0.,0.));
#5612=DIRECTION('center_axis',(0.,0.,-1.));
#5613=DIRECTION('ref_axis',(1.,0.,0.));
#5614=DIRECTION('',(0.,0.,1.));
#5615=DIRECTION('center_axis',(0.,0.,-1.));
#5616=DIRECTION('ref_axis',(1.,0.,0.));
#5617=DIRECTION('center_axis',(0.,0.,1.));
#5618=DIRECTION('ref_axis',(1.,0.,0.));
#5619=DIRECTION('center_axis',(0.,0.,1.));
#5620=DIRECTION('ref_axis',(1.,0.,0.));
#5621=DIRECTION('',(0.,0.,1.));
#5622=DIRECTION('center_axis',(0.,0.,1.));
#5623=DIRECTION('ref_axis',(1.,0.,0.));
#5624=DIRECTION('center_axis',(0.,0.,1.));
#5625=DIRECTION('ref_axis',(1.,0.,0.));
#5626=DIRECTION('center_axis',(0.,0.,1.));
#5627=DIRECTION('ref_axis',(1.,0.,0.));
#5628=DIRECTION('center_axis',(0.,0.,1.));
#5629=DIRECTION('ref_axis',(1.,0.,0.));
#5630=DIRECTION('center_axis',(0.,0.,1.));
#5631=DIRECTION('ref_axis',(1.,0.,0.));
#5632=DIRECTION('',(-1.,0.,0.));
#5633=DIRECTION('center_axis',(0.,0.,1.));
#5634=DIRECTION('ref_axis',(1.,0.,0.));
#5635=DIRECTION('center_axis',(0.,0.,1.));
#5636=DIRECTION('ref_axis',(1.,0.,0.));
#5637=DIRECTION('center_axis',(0.,0.,1.));
#5638=DIRECTION('ref_axis',(1.,0.,0.));
#5639=DIRECTION('',(0.,0.,-1.));
#5640=DIRECTION('',(0.,0.,1.));
#5641=DIRECTION('',(0.,0.,1.));
#5642=DIRECTION('center_axis',(0.,0.,-1.));
#5643=DIRECTION('ref_axis',(1.,0.,0.));
#5644=DIRECTION('center_axis',(0.,0.,1.));
#5645=DIRECTION('ref_axis',(1.,0.,0.));
#5646=DIRECTION('center_axis',(0.,0.,1.));
#5647=DIRECTION('ref_axis',(1.,0.,0.));
#5648=DIRECTION('',(0.,0.,1.));
#5649=DIRECTION('center_axis',(0.,0.,-1.));
#5650=DIRECTION('ref_axis',(1.,0.,0.));
#5651=DIRECTION('center_axis',(0.,0.,1.));
#5652=DIRECTION('ref_axis',(1.,0.,0.));
#5653=DIRECTION('center_axis',(0.,0.,1.));
#5654=DIRECTION('ref_axis',(1.,0.,0.));
#5655=DIRECTION('center_axis',(0.,0.,1.));
#5656=DIRECTION('ref_axis',(1.,0.,0.));
#5657=DIRECTION('',(0.,0.,1.));
#5658=DIRECTION('center_axis',(0.,0.,-1.));
#5659=DIRECTION('ref_axis',(1.,0.,0.));
#5660=DIRECTION('center_axis',(0.,0.,1.));
#5661=DIRECTION('ref_axis',(1.,0.,0.));
#5662=DIRECTION('center_axis',(0.,0.,1.));
#5663=DIRECTION('ref_axis',(1.,0.,0.));
#5664=DIRECTION('center_axis',(0.,0.,1.));
#5665=DIRECTION('ref_axis',(1.,0.,0.));
#5666=DIRECTION('',(0.,0.,1.));
#5667=DIRECTION('center_axis',(0.,0.,-1.));
#5668=DIRECTION('ref_axis',(1.,0.,0.));
#5669=DIRECTION('center_axis',(0.,0.,1.));
#5670=DIRECTION('ref_axis',(1.,0.,0.));
#5671=DIRECTION('center_axis',(0.,0.,1.));
#5672=DIRECTION('ref_axis',(1.,0.,0.));
#5673=DIRECTION('center_axis',(0.,0.,1.));
#5674=DIRECTION('ref_axis',(1.,0.,0.));
#5675=DIRECTION('',(0.,0.,1.));
#5676=DIRECTION('center_axis',(0.,0.,-1.));
#5677=DIRECTION('ref_axis',(1.,0.,0.));
#5678=DIRECTION('center_axis',(0.,0.,1.));
#5679=DIRECTION('ref_axis',(1.,0.,0.));
#5680=DIRECTION('center_axis',(0.,0.,1.));
#5681=DIRECTION('ref_axis',(1.,0.,0.));
#5682=DIRECTION('center_axis',(0.,0.,1.));
#5683=DIRECTION('ref_axis',(1.,0.,0.));
#5684=DIRECTION('',(0.,0.,1.));
#5685=DIRECTION('center_axis',(0.,0.,-1.));
#5686=DIRECTION('ref_axis',(1.,0.,0.));
#5687=DIRECTION('center_axis',(0.,0.,1.));
#5688=DIRECTION('ref_axis',(1.,0.,0.));
#5689=DIRECTION('center_axis',(0.,1.,0.));
#5690=DIRECTION('ref_axis',(1.,0.,0.));
#5691=DIRECTION('center_axis',(0.,1.,0.));
#5692=DIRECTION('ref_axis',(1.,0.,0.));
#5693=DIRECTION('center_axis',(0.,1.,0.));
#5694=DIRECTION('ref_axis',(1.,0.,0.));
#5695=DIRECTION('center_axis',(0.,1.,0.));
#5696=DIRECTION('ref_axis',(1.,0.,0.));
#5697=DIRECTION('center_axis',(0.,0.,1.));
#5698=DIRECTION('ref_axis',(1.,0.,0.));
#5699=DIRECTION('',(0.,-1.,0.));
#5700=DIRECTION('center_axis',(0.,0.,1.));
#5701=DIRECTION('ref_axis',(1.,0.,0.));
#5702=DIRECTION('center_axis',(0.,0.,1.));
#5703=DIRECTION('ref_axis',(1.,0.,0.));
#5704=DIRECTION('',(0.,1.,0.));
#5705=DIRECTION('center_axis',(0.,0.,1.));
#5706=DIRECTION('ref_axis',(1.,0.,0.));
#5707=DIRECTION('center_axis',(0.,0.,1.));
#5708=DIRECTION('ref_axis',(-1.,1.22464679914735E-16,0.));
#5709=DIRECTION('center_axis',(0.,-0.707106781186548,-0.707106781186547));
#5710=DIRECTION('ref_axis',(0.,0.707106781186547,-0.707106781186548));
#5711=DIRECTION('center_axis',(0.,0.707106781186548,-0.707106781186547));
#5712=DIRECTION('ref_axis',(0.,0.707106781186547,0.707106781186548));
#5713=DIRECTION('center_axis',(0.,0.,1.));
#5714=DIRECTION('ref_axis',(1.,0.,0.));
#5715=DIRECTION('center_axis',(0.,0.707106781186548,-0.707106781186547));
#5716=DIRECTION('ref_axis',(0.,0.707106781186547,0.707106781186548));
#5717=DIRECTION('center_axis',(0.,-0.707106781186548,-0.707106781186547));
#5718=DIRECTION('ref_axis',(0.,0.707106781186547,-0.707106781186548));
#5719=DIRECTION('center_axis',(0.,0.,1.));
#5720=DIRECTION('ref_axis',(1.,0.,0.));
#5721=DIRECTION('center_axis',(0.,0.707106781186548,0.707106781186547));
#5722=DIRECTION('ref_axis',(0.,0.707106781186547,-0.707106781186548));
#5723=DIRECTION('',(0.,0.,1.));
#5724=DIRECTION('center_axis',(0.,0.,-1.));
#5725=DIRECTION('ref_axis',(1.,0.,0.));
#5726=DIRECTION('center_axis',(0.,-0.707106781186548,0.707106781186547));
#5727=DIRECTION('ref_axis',(0.,0.707106781186547,0.707106781186548));
#5728=DIRECTION('center_axis',(0.,1.,0.));
#5729=DIRECTION('ref_axis',(1.,0.,0.));
#5730=DIRECTION('',(0.,1.,0.));
#5731=DIRECTION('',(0.,1.,0.));
#5732=DIRECTION('center_axis',(0.,1.,0.));
#5733=DIRECTION('ref_axis',(1.,0.,0.));
#5734=DIRECTION('',(0.,1.,0.));
#5735=DIRECTION('center_axis',(1.,0.,0.));
#5736=DIRECTION('ref_axis',(0.,0.,-1.));
#5737=DIRECTION('',(1.,0.,0.));
#5738=DIRECTION('center_axis',(-1.,0.,0.));
#5739=DIRECTION('ref_axis',(0.,0.,-1.));
#5740=DIRECTION('center_axis',(1.,0.,0.));
#5741=DIRECTION('ref_axis',(0.,0.,-1.));
#5742=DIRECTION('center_axis',(1.,0.,0.));
#5743=DIRECTION('ref_axis',(0.,0.,-1.));
#5744=DIRECTION('',(1.,0.,0.));
#5745=DIRECTION('center_axis',(1.,0.,0.));
#5746=DIRECTION('ref_axis',(0.,0.,-1.));
#5747=DIRECTION('center_axis',(0.,0.,1.));
#5748=DIRECTION('ref_axis',(1.,0.,0.));
#5749=DIRECTION('',(-1.,0.,0.));
#5750=DIRECTION('center_axis',(0.,0.,1.));
#5751=DIRECTION('ref_axis',(1.,0.,0.));
#5752=DIRECTION('center_axis',(0.,0.,1.));
#5753=DIRECTION('ref_axis',(1.,0.,0.));
#5754=DIRECTION('',(1.,0.,0.));
#5755=DIRECTION('center_axis',(0.,0.,1.));
#5756=DIRECTION('ref_axis',(1.,0.,0.));
#5757=DIRECTION('center_axis',(0.,0.,1.));
#5758=DIRECTION('ref_axis',(1.,0.,0.));
#5759=DIRECTION('',(0.,-1.,0.));
#5760=DIRECTION('center_axis',(0.,0.,1.));
#5761=DIRECTION('ref_axis',(1.,0.,0.));
#5762=DIRECTION('center_axis',(0.,0.,1.));
#5763=DIRECTION('ref_axis',(1.,0.,0.));
#5764=DIRECTION('center_axis',(0.707106781186547,0.,0.707106781186548));
#5765=DIRECTION('ref_axis',(0.707106781186548,0.,-0.707106781186547));
#5766=DIRECTION('center_axis',(-0.707106781186547,0.,0.707106781186548));
#5767=DIRECTION('ref_axis',(0.707106781186548,0.,0.707106781186547));
#5768=DIRECTION('center_axis',(0.,0.,1.));
#5769=DIRECTION('ref_axis',(1.,0.,0.));
#5770=DIRECTION('center_axis',(-0.707106781186547,0.,0.707106781186548));
#5771=DIRECTION('ref_axis',(0.707106781186548,0.,0.707106781186547));
#5772=DIRECTION('center_axis',(0.707106781186547,0.,0.707106781186548));
#5773=DIRECTION('ref_axis',(0.707106781186548,0.,-0.707106781186547));
#5774=DIRECTION('center_axis',(0.,0.,1.));
#5775=DIRECTION('ref_axis',(1.,0.,0.));
#5776=DIRECTION('center_axis',(0.,0.,1.));
#5777=DIRECTION('ref_axis',(1.,0.,0.));
#5778=DIRECTION('',(0.,0.,1.));
#5779=DIRECTION('center_axis',(0.707106781186547,0.,-0.707106781186548));
#5780=DIRECTION('ref_axis',(0.707106781186548,0.,0.707106781186547));
#5781=DIRECTION('center_axis',(-0.707106781186547,0.,-0.707106781186548));
#5782=DIRECTION('ref_axis',(0.707106781186548,0.,-0.707106781186547));
#5783=DIRECTION('',(0.,0.,-1.));
#5784=DIRECTION('',(0.,0.,1.));
#5785=DIRECTION('center_axis',(-0.707106781186547,0.,-0.707106781186548));
#5786=DIRECTION('ref_axis',(0.707106781186548,0.,-0.707106781186547));
#5787=DIRECTION('center_axis',(0.707106781186547,0.,-0.707106781186548));
#5788=DIRECTION('ref_axis',(0.707106781186548,0.,0.707106781186547));
#5789=DIRECTION('center_axis',(1.,0.,0.));
#5790=DIRECTION('ref_axis',(0.,0.,-1.));
#5791=DIRECTION('center_axis',(1.,0.,0.));
#5792=DIRECTION('ref_axis',(0.,0.,-1.));
#5793=DIRECTION('center_axis',(1.,0.,0.));
#5794=DIRECTION('ref_axis',(0.,0.,-1.));
#5795=DIRECTION('center_axis',(1.,0.,0.));
#5796=DIRECTION('ref_axis',(0.,0.,-1.));
#5797=DIRECTION('center_axis',(1.,0.,0.));
#5798=DIRECTION('ref_axis',(0.,0.,-1.));
#5799=DIRECTION('',(1.,0.,0.));
#5800=DIRECTION('center_axis',(1.,0.,0.));
#5801=DIRECTION('ref_axis',(0.,0.,-1.));
#5802=DIRECTION('',(1.,0.,0.));
#5803=DIRECTION('center_axis',(1.,0.,0.));
#5804=DIRECTION('ref_axis',(0.,0.,-1.));
#5805=DIRECTION('center_axis',(1.,0.,0.));
#5806=DIRECTION('ref_axis',(0.,0.,-1.));
#5807=DIRECTION('center_axis',(0.,0.,1.));
#5808=DIRECTION('ref_axis',(1.,0.,0.));
#5809=DIRECTION('center_axis',(0.,0.,1.));
#5810=DIRECTION('ref_axis',(1.,0.,0.));
#5811=DIRECTION('',(0.,0.,1.));
#5812=DIRECTION('center_axis',(0.,0.,1.));
#5813=DIRECTION('ref_axis',(1.,0.,0.));
#5814=DIRECTION('center_axis',(0.,0.,1.));
#5815=DIRECTION('ref_axis',(1.,0.,0.));
#5816=DIRECTION('center_axis',(0.,0.,-1.));
#5817=DIRECTION('ref_axis',(1.,0.,0.));
#5818=DIRECTION('center_axis',(0.,0.,1.));
#5819=DIRECTION('ref_axis',(1.,0.,0.));
#5820=DIRECTION('center_axis',(0.,0.,1.));
#5821=DIRECTION('ref_axis',(1.,0.,0.));
#5822=DIRECTION('center_axis',(0.,0.,1.));
#5823=DIRECTION('ref_axis',(1.,0.,0.));
#5824=DIRECTION('center_axis',(0.,0.,1.));
#5825=DIRECTION('ref_axis',(1.,0.,0.));
#5826=DIRECTION('',(0.,0.,1.));
#5827=DIRECTION('center_axis',(0.,0.,1.));
#5828=DIRECTION('ref_axis',(1.,0.,0.));
#5829=DIRECTION('',(0.,0.,1.));
#5830=DIRECTION('center_axis',(0.,0.,-1.));
#5831=DIRECTION('ref_axis',(1.,0.,0.));
#5832=DIRECTION('center_axis',(0.,0.,1.));
#5833=DIRECTION('ref_axis',(1.,0.,0.));
#5834=DIRECTION('center_axis',(0.,0.,1.));
#5835=DIRECTION('ref_axis',(1.,0.,0.));
#5836=DIRECTION('',(0.,0.,-1.));
#5837=DIRECTION('center_axis',(0.,0.,1.));
#5838=DIRECTION('ref_axis',(1.,0.,0.));
#5839=DIRECTION('center_axis',(0.,0.,1.));
#5840=DIRECTION('ref_axis',(1.,0.,0.));
#5841=DIRECTION('center_axis',(0.,0.,-1.));
#5842=DIRECTION('ref_axis',(1.,0.,0.));
#5843=DIRECTION('center_axis',(0.,0.,1.));
#5844=DIRECTION('ref_axis',(1.,0.,0.));
#5845=DIRECTION('center_axis',(0.,0.,1.));
#5846=DIRECTION('ref_axis',(1.,0.,0.));
#5847=DIRECTION('center_axis',(0.,0.,1.));
#5848=DIRECTION('ref_axis',(1.,0.,0.));
#5849=DIRECTION('',(0.,0.,1.));
#5850=DIRECTION('center_axis',(0.,0.,-1.));
#5851=DIRECTION('ref_axis',(1.,0.,0.));
#5852=DIRECTION('center_axis',(0.,0.,1.));
#5853=DIRECTION('ref_axis',(1.,0.,0.));
#5854=DIRECTION('',(0.,0.,1.));
#5855=DIRECTION('center_axis',(0.,0.,1.));
#5856=DIRECTION('ref_axis',(1.,0.,0.));
#5857=DIRECTION('center_axis',(0.,0.,1.));
#5858=DIRECTION('ref_axis',(1.,0.,0.));
#5859=DIRECTION('center_axis',(0.,0.,1.));
#5860=DIRECTION('ref_axis',(1.,0.,0.));
#5861=DIRECTION('center_axis',(0.,0.,1.));
#5862=DIRECTION('ref_axis',(1.,0.,0.));
#5863=DIRECTION('',(0.,0.,1.));
#5864=DIRECTION('center_axis',(0.,0.,-1.));
#5865=DIRECTION('ref_axis',(1.,0.,0.));
#5866=DIRECTION('center_axis',(0.,0.,1.));
#5867=DIRECTION('ref_axis',(1.,0.,0.));
#5868=DIRECTION('center_axis',(0.,0.,1.));
#5869=DIRECTION('ref_axis',(1.,0.,0.));
#5870=DIRECTION('center_axis',(0.,0.,1.));
#5871=DIRECTION('ref_axis',(1.,0.,0.));
#5872=DIRECTION('',(0.,0.,1.));
#5873=DIRECTION('center_axis',(0.,0.,1.));
#5874=DIRECTION('ref_axis',(1.,0.,0.));
#5875=DIRECTION('center_axis',(0.,0.,1.));
#5876=DIRECTION('ref_axis',(1.,0.,0.));
#5877=DIRECTION('center_axis',(0.,0.,1.));
#5878=DIRECTION('ref_axis',(1.,0.,0.));
#5879=DIRECTION('',(0.,0.,-1.));
#5880=DIRECTION('',(0.,0.,-1.));
#5881=DIRECTION('center_axis',(0.,0.,1.));
#5882=DIRECTION('ref_axis',(1.,0.,0.));
#5883=DIRECTION('center_axis',(0.,0.,1.));
#5884=DIRECTION('ref_axis',(1.,0.,0.));
#5885=DIRECTION('center_axis',(0.,0.,1.));
#5886=DIRECTION('ref_axis',(1.,0.,0.));
#7009=CARTESIAN_POINT('',(0.,0.,0.));
#7010=CARTESIAN_POINT('Origin',(-4.,0.,0.9));
#7011=CARTESIAN_POINT('',(-4.165,-2.02066721859313E-17,1.));
#7012=CARTESIAN_POINT('Origin',(-4.,0.,1.));
#7013=CARTESIAN_POINT('',(-4.165,-3.78589117085946E-17,1.615));
#7014=CARTESIAN_POINT('',(-4.165,-2.02066721859313E-17,0.9));
#7015=CARTESIAN_POINT('',(-4.,-0.165,1.63516919445621));
#7016=CARTESIAN_POINT('Ctrl Pts',(-4.,-0.165,1.63516919445621));
#7017=CARTESIAN_POINT('Ctrl Pts',(-4.02080740660683,-0.165,1.63516919445621));
#7018=CARTESIAN_POINT('Ctrl Pts',(-4.0429430103202,-0.160824823566189,1.63409071616177));
#7019=CARTESIAN_POINT('Ctrl Pts',(-4.08356969606673,-0.14396122454405,1.63024260952261));
#7020=CARTESIAN_POINT('Ctrl Pts',(-4.10206824127575,-0.131276996515812,
1.62753363614987));
#7021=CARTESIAN_POINT('Ctrl Pts',(-4.13127524440319,-0.102069993388373,
1.62248518534955));
#7022=CARTESIAN_POINT('Ctrl Pts',(-4.14396083991376,-0.0835707156017109,
1.61981093112785));
#7023=CARTESIAN_POINT('Ctrl Pts',(-4.16082543577155,-0.0429414425249984,
1.61604293526104));
#7024=CARTESIAN_POINT('Ctrl Pts',(-4.165,-0.0208049103060176,1.615));
#7025=CARTESIAN_POINT('Ctrl Pts',(-4.165,1.38777878078145E-17,1.615));
#7026=CARTESIAN_POINT('Ctrl Pts',(-4.165,-1.73472347597681E-17,1.615));
#7027=CARTESIAN_POINT('Ctrl Pts',(-4.165,0.0208049103060176,1.615));
#7028=CARTESIAN_POINT('Ctrl Pts',(-4.16082543577155,0.0429414425249979,
1.61604293526104));
#7029=CARTESIAN_POINT('Ctrl Pts',(-4.14396083991376,0.0835707156017106,
1.61981093112785));
#7030=CARTESIAN_POINT('Ctrl Pts',(-4.13127524440319,0.102069993388373,1.62248518534955));
#7031=CARTESIAN_POINT('Ctrl Pts',(-4.10206824127575,0.131276996515812,1.62753363614987));
#7032=CARTESIAN_POINT('Ctrl Pts',(-4.08356969606673,0.14396122454405,1.63024260952261));
#7033=CARTESIAN_POINT('Ctrl Pts',(-4.0429430103202,0.160824823566189,1.63409071616177));
#7034=CARTESIAN_POINT('Ctrl Pts',(-4.02080740660683,0.165,1.63516919445621));
#7035=CARTESIAN_POINT('Ctrl Pts',(-3.97919259339316,0.165,1.63516919445621));
#7036=CARTESIAN_POINT('Ctrl Pts',(-3.9570569896798,0.160824823566189,1.63409071616177));
#7037=CARTESIAN_POINT('Ctrl Pts',(-3.91643030393327,0.143961224544049,1.63024260952261));
#7038=CARTESIAN_POINT('Ctrl Pts',(-3.89793175872425,0.131276996515812,1.62753363614987));
#7039=CARTESIAN_POINT('Ctrl Pts',(-3.86872475559681,0.102069993388373,1.62248518534955));
#7040=CARTESIAN_POINT('Ctrl Pts',(-3.85603916008624,0.0835707156017107,
1.61981093112785));
#7041=CARTESIAN_POINT('Ctrl Pts',(-3.83917456422845,0.0429414425249981,
1.61604293526104));
#7042=CARTESIAN_POINT('Ctrl Pts',(-3.835,0.0208049103060177,1.615));
#7043=CARTESIAN_POINT('Ctrl Pts',(-3.835,-0.0208049103060176,1.615));
#7044=CARTESIAN_POINT('Ctrl Pts',(-3.83917456422845,-0.042941442524998,
1.61604293526104));
#7045=CARTESIAN_POINT('Ctrl Pts',(-3.85603916008624,-0.0835707156017107,
1.61981093112785));
#7046=CARTESIAN_POINT('Ctrl Pts',(-3.86872475559681,-0.102069993388373,
1.62248518534955));
#7047=CARTESIAN_POINT('Ctrl Pts',(-3.89793175872425,-0.131276996515812,
1.62753363614987));
#7048=CARTESIAN_POINT('Ctrl Pts',(-3.91643030393327,-0.143961224544049,
1.63024260952261));
#7049=CARTESIAN_POINT('Ctrl Pts',(-3.9570569896798,-0.160824823566189,1.63409071616177));
#7050=CARTESIAN_POINT('Ctrl Pts',(-3.97919259339316,-0.165,1.63516919445621));
#7051=CARTESIAN_POINT('Ctrl Pts',(-4.,-0.165,1.63516919445621));
#7052=CARTESIAN_POINT('Origin',(4.,0.,0.9));
#7053=CARTESIAN_POINT('',(3.835,-2.02066721859313E-17,1.));
#7054=CARTESIAN_POINT('Origin',(4.,0.,1.));
#7055=CARTESIAN_POINT('',(3.835,-2.02066721859313E-17,2.1));
#7056=CARTESIAN_POINT('',(3.835,-2.02066721859313E-17,0.9));
#7057=CARTESIAN_POINT('Origin',(4.,0.,2.1));
#7058=CARTESIAN_POINT('Origin',(4.,0.,2.1));
#7059=CARTESIAN_POINT('Origin',(-2.05060966544099,-2.05060966544099,1.3));
#7060=CARTESIAN_POINT('',(-2.21560966544099,-2.05060966544099,1.4));
#7061=CARTESIAN_POINT('Origin',(-2.05060966544099,-2.05060966544099,1.4));
#7062=CARTESIAN_POINT('',(-2.21560966544099,-2.05060966544099,2.7));
#7063=CARTESIAN_POINT('',(-2.21560966544099,-2.05060966544099,1.3));
#7064=CARTESIAN_POINT('Origin',(-2.05060966544099,-2.05060966544099,2.7));
#7065=CARTESIAN_POINT('Origin',(-2.05060966544099,-2.05060966544099,2.7));
#7066=CARTESIAN_POINT('Origin',(-2.05060966544099,2.05060966544099,1.3));
#7067=CARTESIAN_POINT('',(-2.21560966544099,2.05060966544099,1.4));
#7068=CARTESIAN_POINT('Origin',(-2.05060966544099,2.05060966544099,1.4));
#7069=CARTESIAN_POINT('',(-2.21560966544099,2.05060966544099,2.7));
#7070=CARTESIAN_POINT('',(-2.21560966544099,2.05060966544099,1.3));
#7071=CARTESIAN_POINT('Origin',(-2.05060966544099,2.05060966544099,2.7));
#7072=CARTESIAN_POINT('Origin',(-2.05060966544099,2.05060966544099,2.7));
#7073=CARTESIAN_POINT('Origin',(2.05060966544099,2.05060966544099,1.3));
#7074=CARTESIAN_POINT('',(1.88560966544099,2.05060966544099,1.4));
#7075=CARTESIAN_POINT('Origin',(2.05060966544099,2.05060966544099,1.4));
#7076=CARTESIAN_POINT('',(1.88560966544099,2.05060966544099,2.7));
#7077=CARTESIAN_POINT('',(1.88560966544099,2.05060966544099,1.3));
#7078=CARTESIAN_POINT('Origin',(2.05060966544099,2.05060966544099,2.7));
#7079=CARTESIAN_POINT('Origin',(2.05060966544099,2.05060966544099,2.7));
#7080=CARTESIAN_POINT('Origin',(2.05060966544099,-2.05060966544099,1.3));
#7081=CARTESIAN_POINT('',(1.88560966544099,-2.05060966544099,1.4));
#7082=CARTESIAN_POINT('Origin',(2.05060966544099,-2.05060966544099,1.4));
#7083=CARTESIAN_POINT('',(1.88560966544099,-2.05060966544099,2.7));
#7084=CARTESIAN_POINT('',(1.88560966544099,-2.05060966544099,1.3));
#7085=CARTESIAN_POINT('Origin',(2.05060966544099,-2.05060966544099,2.7));
#7086=CARTESIAN_POINT('Origin',(2.05060966544099,-2.05060966544099,2.7));
#7087=CARTESIAN_POINT('Origin',(0.,0.,1.4));
#7088=CARTESIAN_POINT('',(-2.24,-2.74320883009007E-16,1.4));
#7089=CARTESIAN_POINT('Origin',(0.,0.,1.4));
#7090=CARTESIAN_POINT('',(-2.24,-2.74320883009007E-16,1.51));
#7091=CARTESIAN_POINT('',(-2.24,-2.74320883009007E-16,1.4));
#7092=CARTESIAN_POINT('Origin',(0.,0.,1.51));
#7093=CARTESIAN_POINT('Origin',(0.,0.,1.4));
#7094=CARTESIAN_POINT('',(-2.46,-3.01263112590249E-16,1.4));
#7095=CARTESIAN_POINT('Origin',(0.,0.,1.4));
#7096=CARTESIAN_POINT('',(-2.46,-3.01263112590249E-16,1.51));
#7097=CARTESIAN_POINT('',(-2.46,-3.01263112590249E-16,1.4));
#7098=CARTESIAN_POINT('Origin',(0.,0.,1.51));
#7099=CARTESIAN_POINT('Origin',(0.,0.,1.51));
#7100=CARTESIAN_POINT('Origin',(0.,0.,1.4));
#7101=CARTESIAN_POINT('',(-3.31,-4.05358090517774E-16,1.4));
#7102=CARTESIAN_POINT('Origin',(0.,0.,1.4));
#7103=CARTESIAN_POINT('Origin',(-6.38378239159465E-16,-3.4,3.5));
#7104=CARTESIAN_POINT('',(0.184661853126193,-3.5,3.5));
#7105=CARTESIAN_POINT('',(-0.184661853126194,-3.5,3.5));
#7106=CARTESIAN_POINT('',(-3.19189119579733E-16,-3.5,3.5));
#7107=CARTESIAN_POINT('',(-0.210000000000001,-3.4,3.5));
#7108=CARTESIAN_POINT('Origin',(-6.2456986756515E-16,-3.4,3.5));
#7109=CARTESIAN_POINT('Origin',(-6.2456986756515E-16,-3.4,3.5));
#7110=CARTESIAN_POINT('Origin',(-6.2456986756515E-16,-3.4,3.5));
#7111=CARTESIAN_POINT('',(0.184661853126193,-3.5,3.55964005336244));
#7112=CARTESIAN_POINT('',(0.184661853126193,-3.5,3.5));
#7113=CARTESIAN_POINT('',(-0.184661853126194,-3.5,3.55964005336244));
#7114=CARTESIAN_POINT('Ctrl Pts',(-0.184661853126194,-3.5,3.55964005336244));
#7115=CARTESIAN_POINT('Ctrl Pts',(-0.174800846718384,-3.51820951716955,
3.56240057663217));
#7116=CARTESIAN_POINT('Ctrl Pts',(-0.162284556957793,-3.53470029114056,
3.56564880027768));
#7117=CARTESIAN_POINT('Ctrl Pts',(-0.129946422600616,-3.56703842549773,
3.57282972708545));
#7118=CARTESIAN_POINT('Ctrl Pts',(-0.106445900548852,-3.58317393160533,
3.57717919558841));
#7119=CARTESIAN_POINT('Ctrl Pts',(-0.054753956552258,-3.60465928779521,
3.58330402961894));
#7120=CARTESIAN_POINT('Ctrl Pts',(-0.0265493609398035,-3.61,3.585));
#7121=CARTESIAN_POINT('Ctrl Pts',(0.0265493609398022,-3.61,3.585));
#7122=CARTESIAN_POINT('Ctrl Pts',(0.0547539565522566,-3.60465928779521,
3.58330402961894));
#7123=CARTESIAN_POINT('Ctrl Pts',(0.106445900548851,-3.58317393160533,3.57717919558841));
#7124=CARTESIAN_POINT('Ctrl Pts',(0.129946422600615,-3.56703842549773,3.57282972708545));
#7125=CARTESIAN_POINT('Ctrl Pts',(0.162284556957791,-3.53470029114056,3.56564880027768));
#7126=CARTESIAN_POINT('Ctrl Pts',(0.174800846718383,-3.51820951716955,3.56240057663217));
#7127=CARTESIAN_POINT('Ctrl Pts',(0.184661853126193,-3.5,3.55964005336244));
#7128=CARTESIAN_POINT('',(-0.184661853126194,-3.5,3.5));
#7129=CARTESIAN_POINT('',(-0.210000000000001,-3.4,5.));
#7130=CARTESIAN_POINT('',(-0.210000000000001,-3.4,3.5));
#7131=CARTESIAN_POINT('Origin',(-6.2456986756515E-16,-3.4,5.));
#7132=CARTESIAN_POINT('Origin',(2.94448637286709,1.7,3.5));
#7133=CARTESIAN_POINT('',(2.73448637286709,1.7,3.5));
#7134=CARTESIAN_POINT('Origin',(2.94448637286709,1.7,3.5));
#7135=CARTESIAN_POINT('',(2.73448637286709,1.7,5.));
#7136=CARTESIAN_POINT('',(2.73448637286709,1.7,3.5));
#7137=CARTESIAN_POINT('Origin',(2.94448637286709,1.7,5.));
#7138=CARTESIAN_POINT('Origin',(2.94448637286709,1.7,3.5));
#7139=CARTESIAN_POINT('Origin',(2.0818995585505E-16,3.4,3.5));
#7140=CARTESIAN_POINT('',(-0.21,3.4,3.5));
#7141=CARTESIAN_POINT('Origin',(2.0818995585505E-16,3.4,3.5));
#7142=CARTESIAN_POINT('',(-0.21,3.4,5.));
#7143=CARTESIAN_POINT('',(-0.21,3.4,3.5));
#7144=CARTESIAN_POINT('Origin',(2.0818995585505E-16,3.4,5.));
#7145=CARTESIAN_POINT('Origin',(2.22044604925031E-16,3.4,3.5));
#7146=CARTESIAN_POINT('Origin',(-2.94448637286709,1.7,3.5));
#7147=CARTESIAN_POINT('',(-3.15448637286709,1.7,3.5));
#7148=CARTESIAN_POINT('Origin',(-2.94448637286709,1.7,3.5));
#7149=CARTESIAN_POINT('',(-3.15448637286709,1.7,5.));
#7150=CARTESIAN_POINT('',(-3.15448637286709,1.7,3.5));
#7151=CARTESIAN_POINT('Origin',(-2.94448637286709,1.7,5.));
#7152=CARTESIAN_POINT('Origin',(-2.94448637286709,1.7,3.5));
#7153=CARTESIAN_POINT('Origin',(-2.94448637286709,-1.7,3.5));
#7154=CARTESIAN_POINT('',(-3.15448637286709,-1.7,3.5));
#7155=CARTESIAN_POINT('Origin',(-2.94448637286709,-1.7,3.5));
#7156=CARTESIAN_POINT('',(-3.15448637286709,-1.7,5.));
#7157=CARTESIAN_POINT('',(-3.15448637286709,-1.7,3.5));
#7158=CARTESIAN_POINT('Origin',(-2.94448637286709,-1.7,5.));
#7159=CARTESIAN_POINT('Origin',(-2.94448637286709,-1.7,3.5));
#7160=CARTESIAN_POINT('Origin',(2.94448637286709,-1.7,3.5));
#7161=CARTESIAN_POINT('',(2.73448637286709,-1.7,3.5));
#7162=CARTESIAN_POINT('Origin',(2.94448637286709,-1.7,3.5));
#7163=CARTESIAN_POINT('',(2.73448637286709,-1.7,5.));
#7164=CARTESIAN_POINT('',(2.73448637286709,-1.7,3.5));
#7165=CARTESIAN_POINT('Origin',(2.94448637286709,-1.7,5.));
#7166=CARTESIAN_POINT('Origin',(2.94448637286709,-1.7,3.5));
#7167=CARTESIAN_POINT('Origin',(0.,-3.5,2.9));
#7168=CARTESIAN_POINT('',(-0.685,-3.5,2.9));
#7169=CARTESIAN_POINT('Origin',(0.,-3.5,2.9));
#7170=CARTESIAN_POINT('Origin',(0.,-3.5,2.9));
#7171=CARTESIAN_POINT('',(-0.2,-3.5,2.9));
#7172=CARTESIAN_POINT('Origin',(0.,-3.5,2.9));
#7173=CARTESIAN_POINT('Origin',(0.,-2.,2.8));
#7174=CARTESIAN_POINT('',(-0.173205080756888,-1.9,2.8));
#7175=CARTESIAN_POINT('',(-0.173205080756888,-2.1,2.8));
#7176=CARTESIAN_POINT('',(-0.173205080756888,-3.6,2.8));
#7177=CARTESIAN_POINT('Origin',(0.,-2.,2.8));
#7178=CARTESIAN_POINT('Origin',(0.,-2.,2.8));
#7179=CARTESIAN_POINT('',(0.173205080756888,-2.1,2.8));
#7180=CARTESIAN_POINT('',(0.173205080756888,-1.9,2.8));
#7181=CARTESIAN_POINT('',(0.173205080756888,-3.6,2.8));
#7182=CARTESIAN_POINT('Origin',(0.,-2.,2.8));
#7183=CARTESIAN_POINT('Origin',(0.,-2.,2.8));
#7184=CARTESIAN_POINT('',(-0.2,-2.,2.9));
#7185=CARTESIAN_POINT('Origin',(0.,-2.,2.9));
#7186=CARTESIAN_POINT('Origin',(0.,-2.,2.9));
#7187=CARTESIAN_POINT('Origin',(0.,-2.,2.8));
#7188=CARTESIAN_POINT('',(0.2,-2.,2.9));
#7189=CARTESIAN_POINT('Origin',(0.,-2.,2.9));
#7190=CARTESIAN_POINT('Origin',(0.,-2.,2.9));
#7191=CARTESIAN_POINT('Origin',(0.,-2.,2.8));
#7192=CARTESIAN_POINT('Origin',(0.,-2.,2.9));
#7193=CARTESIAN_POINT('',(-0.2,-2.,3.2));
#7194=CARTESIAN_POINT('',(-0.2,-2.,2.8));
#7195=CARTESIAN_POINT('Origin',(0.,-2.,3.2));
#7196=CARTESIAN_POINT('Origin',(0.,-2.,2.9));
#7197=CARTESIAN_POINT('Origin',(0.,-3.6,2.9));
#7198=CARTESIAN_POINT('',(-0.2,-3.6,2.9));
#7199=CARTESIAN_POINT('',(-0.2,-0.565685424949238,2.9));
#7200=CARTESIAN_POINT('',(-0.2,-3.6,2.9));
#7201=CARTESIAN_POINT('Ctrl Pts',(-0.2,-0.565685424949238,2.9));
#7202=CARTESIAN_POINT('Ctrl Pts',(-0.2,-0.565685424949238,2.87467078791842));
#7203=CARTESIAN_POINT('Ctrl Pts',(-0.194898067853762,-0.567565356574251,
2.8477996053073));
#7204=CARTESIAN_POINT('Ctrl Pts',(-0.17443058152527,-0.574186082552466,
2.79858936400846));
#7205=CARTESIAN_POINT('Ctrl Pts',(-0.159074095999941,-0.578813771212596,
2.77623138352532));
#7206=CARTESIAN_POINT('Ctrl Pts',(-0.123776803829002,-0.587374622031365,
2.74093409135438));
#7207=CARTESIAN_POINT('Ctrl Pts',(-0.101415562391481,-0.59188739106068,
2.72557130277668));
#7208=CARTESIAN_POINT('Ctrl Pts',(-0.0521932274441715,-0.598240475886912,
2.70509911583939));
#7209=CARTESIAN_POINT('Ctrl Pts',(-0.0253174643734703,-0.6,2.7));
#7210=CARTESIAN_POINT('Ctrl Pts',(0.0253174643734703,-0.6,2.7));
#7211=CARTESIAN_POINT('Ctrl Pts',(0.0521932274441715,-0.598240475886912,
2.70509911583939));
#7212=CARTESIAN_POINT('Ctrl Pts',(0.101415562391481,-0.59188739106068,2.72557130277668));
#7213=CARTESIAN_POINT('Ctrl Pts',(0.123776803829002,-0.587374622031365,
2.74093409135438));
#7214=CARTESIAN_POINT('Ctrl Pts',(0.159074095999941,-0.578813771212596,
2.77623138352532));
#7215=CARTESIAN_POINT('Ctrl Pts',(0.17443058152527,-0.574186082552466,2.79858936400846));
#7216=CARTESIAN_POINT('Ctrl Pts',(0.194898067853762,-0.567565356574251,
2.8477996053073));
#7217=CARTESIAN_POINT('Ctrl Pts',(0.2,-0.565685424949238,2.87467078791842));
#7218=CARTESIAN_POINT('Ctrl Pts',(0.2,-0.565685424949238,2.92532921208158));
#7219=CARTESIAN_POINT('Ctrl Pts',(0.194898067853762,-0.567565356574251,
2.9522003946927));
#7220=CARTESIAN_POINT('Ctrl Pts',(0.17443058152527,-0.574186082552466,3.00141063599154));
#7221=CARTESIAN_POINT('Ctrl Pts',(0.159074095999941,-0.578813771212596,
3.02376861647468));
#7222=CARTESIAN_POINT('Ctrl Pts',(0.123776803829002,-0.587374622031365,
3.05906590864562));
#7223=CARTESIAN_POINT('Ctrl Pts',(0.101415562391481,-0.59188739106068,3.07442869722332));
#7224=CARTESIAN_POINT('Ctrl Pts',(0.052193227444171,-0.598240475886912,
3.09490088416061));
#7225=CARTESIAN_POINT('Ctrl Pts',(0.0253174643734703,-0.6,3.1));
#7226=CARTESIAN_POINT('Ctrl Pts',(-0.0253174643734703,-0.6,3.1));
#7227=CARTESIAN_POINT('Ctrl Pts',(-0.052193227444171,-0.598240475886912,
3.09490088416061));
#7228=CARTESIAN_POINT('Ctrl Pts',(-0.101415562391481,-0.59188739106068,
3.07442869722332));
#7229=CARTESIAN_POINT('Ctrl Pts',(-0.123776803829002,-0.587374622031365,
3.05906590864562));
#7230=CARTESIAN_POINT('Ctrl Pts',(-0.159074095999941,-0.578813771212596,
3.02376861647468));
#7231=CARTESIAN_POINT('Ctrl Pts',(-0.17443058152527,-0.574186082552466,
3.00141063599154));
#7232=CARTESIAN_POINT('Ctrl Pts',(-0.194898067853762,-0.567565356574251,
2.9522003946927));
#7233=CARTESIAN_POINT('Ctrl Pts',(-0.2,-0.565685424949238,2.92532921208158));
#7234=CARTESIAN_POINT('Ctrl Pts',(-0.2,-0.565685424949238,2.9));
#7235=CARTESIAN_POINT('Origin',(0.,-4.6,2.9));
#7236=CARTESIAN_POINT('',(-0.685,-4.44755831889813,2.9));
#7237=CARTESIAN_POINT('Ctrl Pts',(-0.685,-4.44755831889813,2.9));
#7238=CARTESIAN_POINT('Ctrl Pts',(-0.685,-4.44755831889813,2.98615495576053));
#7239=CARTESIAN_POINT('Ctrl Pts',(-0.667754444280465,-4.4503204226392,3.07795945171461));
#7240=CARTESIAN_POINT('Ctrl Pts',(-0.597806423657171,-4.46025507446226,
3.24668870614449));
#7241=CARTESIAN_POINT('Ctrl Pts',(-0.545111157186078,-4.46727957365527,
3.32362513303949));
#7242=CARTESIAN_POINT('Ctrl Pts',(-0.42362625704472,-4.48043230270009,3.44511003318085));
#7243=CARTESIAN_POINT('Ctrl Pts',(-0.346689345476453,-4.48742111878839,
3.49780618135505));
#7244=CARTESIAN_POINT('Ctrl Pts',(-0.177958434129502,-4.49727390705164,
3.56775484339031));
#7245=CARTESIAN_POINT('Ctrl Pts',(-0.0861533615257771,-4.5,3.585));
#7246=CARTESIAN_POINT('Ctrl Pts',(0.0861533615257768,-4.5,3.585));
#7247=CARTESIAN_POINT('Ctrl Pts',(0.177958434129502,-4.49727390705164,3.56775484339031));
#7248=CARTESIAN_POINT('Ctrl Pts',(0.346689345476453,-4.48742111878839,3.49780618135505));
#7249=CARTESIAN_POINT('Ctrl Pts',(0.42362625704472,-4.48043230270009,3.44511003318085));
#7250=CARTESIAN_POINT('Ctrl Pts',(0.545111157186078,-4.46727957365527,3.32362513303949));
#7251=CARTESIAN_POINT('Ctrl Pts',(0.59780642365717,-4.46025507446226,3.24668870614449));
#7252=CARTESIAN_POINT('Ctrl Pts',(0.667754444280465,-4.4503204226392,3.07795945171461));
#7253=CARTESIAN_POINT('Ctrl Pts',(0.685,-4.44755831889813,2.98615495576053));
#7254=CARTESIAN_POINT('Ctrl Pts',(0.685,-4.44755831889813,2.81384504423947));
#7255=CARTESIAN_POINT('Ctrl Pts',(0.667754444280465,-4.4503204226392,2.72204054828539));
#7256=CARTESIAN_POINT('Ctrl Pts',(0.597806423657171,-4.46025507446226,2.55331129385551));
#7257=CARTESIAN_POINT('Ctrl Pts',(0.545111157186078,-4.46727957365527,2.47637486696051));
#7258=CARTESIAN_POINT('Ctrl Pts',(0.42362625704472,-4.48043230270009,2.35488996681915));
#7259=CARTESIAN_POINT('Ctrl Pts',(0.346689345476454,-4.48742111878839,2.30219381864495));
#7260=CARTESIAN_POINT('Ctrl Pts',(0.177958434129502,-4.49727390705164,2.23224515660969));
#7261=CARTESIAN_POINT('Ctrl Pts',(0.0861533615257774,-4.5,2.215));
#7262=CARTESIAN_POINT('Ctrl Pts',(-0.0861533615257767,-4.5,2.215));
#7263=CARTESIAN_POINT('Ctrl Pts',(-0.177958434129502,-4.49727390705164,
2.23224515660969));
#7264=CARTESIAN_POINT('Ctrl Pts',(-0.346689345476453,-4.48742111878839,
2.30219381864495));
#7265=CARTESIAN_POINT('Ctrl Pts',(-0.423626257044719,-4.48043230270009,
2.35488996681915));
#7266=CARTESIAN_POINT('Ctrl Pts',(-0.545111157186078,-4.46727957365527,
2.47637486696051));
#7267=CARTESIAN_POINT('Ctrl Pts',(-0.59780642365717,-4.46025507446226,2.55331129385551));
#7268=CARTESIAN_POINT('Ctrl Pts',(-0.667754444280465,-4.4503204226392,2.72204054828539));
#7269=CARTESIAN_POINT('Ctrl Pts',(-0.685,-4.44755831889813,2.81384504423947));
#7270=CARTESIAN_POINT('Ctrl Pts',(-0.685,-4.44755831889813,2.9));
#7271=CARTESIAN_POINT('',(-0.685,-4.6,2.9));
#7272=CARTESIAN_POINT('Origin',(-0.1,0.,3.9));
#7273=CARTESIAN_POINT('',(2.46779253585061,0.4,3.9));
#7274=CARTESIAN_POINT('',(2.5,-3.67625427122537E-18,4.3));
#7275=CARTESIAN_POINT('Ctrl Pts',(2.46779253585061,0.4,3.9));
#7276=CARTESIAN_POINT('Ctrl Pts',(2.46779253585061,0.4,3.95031849222446));
#7277=CARTESIAN_POINT('Ctrl Pts',(2.46949065540042,0.389926098864548,4.00393070664371));
#7278=CARTESIAN_POINT('Ctrl Pts',(2.47559507764305,0.3490780234852,4.10245615200085));
#7279=CARTESIAN_POINT('Ctrl Pts',(2.47991004659989,0.318308483288254,4.14737694166098));
#7280=CARTESIAN_POINT('Ctrl Pts',(2.48798680132732,0.247377744540872,4.21830768040837));
#7281=CARTESIAN_POINT('Ctrl Pts',(2.49227754123301,0.202456609487086,4.24907785041389));
#7282=CARTESIAN_POINT('Ctrl Pts',(2.49832635585429,0.103929980260481,4.28992638341895));
#7283=CARTESIAN_POINT('Ctrl Pts',(2.5,0.0503173531062475,4.3));
#7284=CARTESIAN_POINT('Ctrl Pts',(2.5,8.32667268468867E-17,4.3));
#7285=CARTESIAN_POINT('Ctrl Pts',(2.5,2.77555756156289E-17,4.3));
#7286=CARTESIAN_POINT('Ctrl Pts',(2.5,-0.0503173531062473,4.3));
#7287=CARTESIAN_POINT('Ctrl Pts',(2.49832635585429,-0.103929980260481,4.28992638341895));
#7288=CARTESIAN_POINT('Ctrl Pts',(2.49227754123301,-0.202456609487086,4.24907785041389));
#7289=CARTESIAN_POINT('Ctrl Pts',(2.48798680132732,-0.247377744540872,4.21830768040837));
#7290=CARTESIAN_POINT('Ctrl Pts',(2.47991004659989,-0.318308483288254,4.14737694166098));
#7291=CARTESIAN_POINT('Ctrl Pts',(2.47559507764305,-0.3490780234852,4.10245615200085));
#7292=CARTESIAN_POINT('Ctrl Pts',(2.46949065540042,-0.389926098864548,4.00393070664371));
#7293=CARTESIAN_POINT('Ctrl Pts',(2.46779253585061,-0.4,3.95031849222446));
#7294=CARTESIAN_POINT('Ctrl Pts',(2.46779253585061,-0.4,3.84968150777554));
#7295=CARTESIAN_POINT('Ctrl Pts',(2.46949065540042,-0.389926098864548,3.79606929335629));
#7296=CARTESIAN_POINT('Ctrl Pts',(2.47559507764305,-0.3490780234852,3.69754384799915));
#7297=CARTESIAN_POINT('Ctrl Pts',(2.47991004659989,-0.318308483288254,3.65262305833902));
#7298=CARTESIAN_POINT('Ctrl Pts',(2.48798680132732,-0.247377744540872,3.58169231959163));
#7299=CARTESIAN_POINT('Ctrl Pts',(2.49227754123301,-0.202456609487086,3.55092214958611));
#7300=CARTESIAN_POINT('Ctrl Pts',(2.49832635585429,-0.103929980260481,3.51007361658105));
#7301=CARTESIAN_POINT('Ctrl Pts',(2.5,-0.0503173531062475,3.5));
#7302=CARTESIAN_POINT('Ctrl Pts',(2.5,0.0503173531062473,3.5));
#7303=CARTESIAN_POINT('Ctrl Pts',(2.49832635585429,0.103929980260481,3.51007361658105));
#7304=CARTESIAN_POINT('Ctrl Pts',(2.49227754123301,0.202456609487086,3.55092214958611));
#7305=CARTESIAN_POINT('Ctrl Pts',(2.48798680132732,0.247377744540872,3.58169231959163));
#7306=CARTESIAN_POINT('Ctrl Pts',(2.47991004659989,0.318308483288254,3.65262305833902));
#7307=CARTESIAN_POINT('Ctrl Pts',(2.47559507764305,0.3490780234852,3.69754384799915));
#7308=CARTESIAN_POINT('Ctrl Pts',(2.46949065540042,0.389926098864548,3.79606929335629));
#7309=CARTESIAN_POINT('Ctrl Pts',(2.46779253585061,0.4,3.84968150777554));
#7310=CARTESIAN_POINT('Ctrl Pts',(2.46779253585061,0.4,3.9));
#7311=CARTESIAN_POINT('',(3.,4.89858719658941E-17,4.3));
#7312=CARTESIAN_POINT('',(-0.1,-4.89858719658941E-17,4.3));
#7313=CARTESIAN_POINT('Origin',(3.,0.,3.9));
#7314=CARTESIAN_POINT('Origin',(3.,0.,3.9));
#7315=CARTESIAN_POINT('',(3.,-8.38883057415937E-17,4.585));
#7316=CARTESIAN_POINT('Origin',(3.,0.,3.9));
#7317=CARTESIAN_POINT('',(4.5,-8.38883057415937E-17,4.585));
#7318=CARTESIAN_POINT('',(3.,-8.38883057415937E-17,4.585));
#7319=CARTESIAN_POINT('',(4.44755831889813,0.685,3.9));
#7320=CARTESIAN_POINT('Ctrl Pts',(4.44755831889813,0.685,3.9));
#7321=CARTESIAN_POINT('Ctrl Pts',(4.44755831889813,0.685,3.81384504423947));
#7322=CARTESIAN_POINT('Ctrl Pts',(4.4503204226392,0.667754444280465,3.72204054828539));
#7323=CARTESIAN_POINT('Ctrl Pts',(4.46025507446226,0.59780642365717,3.55331129385551));
#7324=CARTESIAN_POINT('Ctrl Pts',(4.46727957365527,0.545111157186078,3.47637486696051));
#7325=CARTESIAN_POINT('Ctrl Pts',(4.48043230270009,0.42362625704472,3.35488996681915));
#7326=CARTESIAN_POINT('Ctrl Pts',(4.48742111878839,0.346689345476453,3.30219381864495));
#7327=CARTESIAN_POINT('Ctrl Pts',(4.49727390705164,0.177958434129502,3.23224515660969));
#7328=CARTESIAN_POINT('Ctrl Pts',(4.5,0.086153361525777,3.215));
#7329=CARTESIAN_POINT('Ctrl Pts',(4.5,-0.0861533615257769,3.215));
#7330=CARTESIAN_POINT('Ctrl Pts',(4.49727390705164,-0.177958434129502,3.23224515660969));
#7331=CARTESIAN_POINT('Ctrl Pts',(4.48742111878839,-0.346689345476453,3.30219381864495));
#7332=CARTESIAN_POINT('Ctrl Pts',(4.48043230270009,-0.42362625704472,3.35488996681915));
#7333=CARTESIAN_POINT('Ctrl Pts',(4.46727957365527,-0.545111157186078,3.47637486696051));
#7334=CARTESIAN_POINT('Ctrl Pts',(4.46025507446226,-0.597806423657171,3.55331129385551));
#7335=CARTESIAN_POINT('Ctrl Pts',(4.4503204226392,-0.667754444280465,3.72204054828539));
#7336=CARTESIAN_POINT('Ctrl Pts',(4.44755831889813,-0.685,3.81384504423947));
#7337=CARTESIAN_POINT('Ctrl Pts',(4.44755831889813,-0.685,3.98615495576053));
#7338=CARTESIAN_POINT('Ctrl Pts',(4.4503204226392,-0.667754444280465,4.0779594517146));
#7339=CARTESIAN_POINT('Ctrl Pts',(4.46025507446226,-0.597806423657171,4.24668870614449));
#7340=CARTESIAN_POINT('Ctrl Pts',(4.46727957365527,-0.545111157186078,4.32362513303949));
#7341=CARTESIAN_POINT('Ctrl Pts',(4.48043230270009,-0.42362625704472,4.44511003318085));
#7342=CARTESIAN_POINT('Ctrl Pts',(4.48742111878839,-0.346689345476454,4.49780618135505));
#7343=CARTESIAN_POINT('Ctrl Pts',(4.49727390705164,-0.177958434129502,4.56775484339031));
#7344=CARTESIAN_POINT('Ctrl Pts',(4.5,-0.0861533615257772,4.585));
#7345=CARTESIAN_POINT('Ctrl Pts',(4.5,-1.38777878078145E-16,4.585));
#7346=CARTESIAN_POINT('Ctrl Pts',(4.5,-8.32667268468867E-17,4.585));
#7347=CARTESIAN_POINT('Ctrl Pts',(4.5,0.086153361525777,4.585));
#7348=CARTESIAN_POINT('Ctrl Pts',(4.49727390705164,0.177958434129502,4.56775484339031));
#7349=CARTESIAN_POINT('Ctrl Pts',(4.48742111878839,0.346689345476453,4.49780618135505));
#7350=CARTESIAN_POINT('Ctrl Pts',(4.48043230270009,0.42362625704472,4.44511003318085));
#7351=CARTESIAN_POINT('Ctrl Pts',(4.46727957365527,0.545111157186078,4.32362513303949));
#7352=CARTESIAN_POINT('Ctrl Pts',(4.46025507446226,0.597806423657171,4.24668870614449));
#7353=CARTESIAN_POINT('Ctrl Pts',(4.4503204226392,0.667754444280465,4.07795945171461));
#7354=CARTESIAN_POINT('Ctrl Pts',(4.44755831889813,0.685,3.98615495576053));
#7355=CARTESIAN_POINT('Ctrl Pts',(4.44755831889813,0.685,3.9));
#7356=CARTESIAN_POINT('Origin',(3.,0.,3.9));
#7357=CARTESIAN_POINT('Origin',(-1.8,0.,2.4));
#7358=CARTESIAN_POINT('',(-1.7,-0.387298334620742,2.4));
#7359=CARTESIAN_POINT('',(-1.9,-0.387298334620742,2.4));
#7360=CARTESIAN_POINT('',(-3.1,-0.387298334620742,2.4));
#7361=CARTESIAN_POINT('Origin',(-1.8,0.,2.4));
#7362=CARTESIAN_POINT('Origin',(-1.8,0.,2.4));
#7363=CARTESIAN_POINT('',(-1.9,0.387298334620742,2.4));
#7364=CARTESIAN_POINT('',(-1.7,0.387298334620742,2.4));
#7365=CARTESIAN_POINT('',(-3.1,0.387298334620742,2.4));
#7366=CARTESIAN_POINT('Origin',(-1.8,0.,2.4));
#7367=CARTESIAN_POINT('Origin',(-1.8,0.,2.4));
#7368=CARTESIAN_POINT('',(-1.6,0.346410161513776,2.4));
#7369=CARTESIAN_POINT('',(-1.6,-0.346410161513776,2.4));
#7370=CARTESIAN_POINT('',(-1.6,0.,2.4));
#7371=CARTESIAN_POINT('Origin',(-1.8,0.,2.4));
#7372=CARTESIAN_POINT('Origin',(-1.8,0.,0.9));
#7373=CARTESIAN_POINT('',(-1.8,-0.4,2.3));
#7374=CARTESIAN_POINT('Origin',(-1.8,0.,2.3));
#7375=CARTESIAN_POINT('Origin',(-1.8,0.,2.3));
#7376=CARTESIAN_POINT('Origin',(-1.8,0.,0.9));
#7377=CARTESIAN_POINT('',(-1.8,0.4,2.3));
#7378=CARTESIAN_POINT('Origin',(-1.8,0.,2.3));
#7379=CARTESIAN_POINT('Origin',(-1.8,0.,2.3));
#7380=CARTESIAN_POINT('Origin',(-1.8,0.,0.9));
#7381=CARTESIAN_POINT('',(-2.2,-4.89858719658941E-17,1.4));
#7382=CARTESIAN_POINT('Origin',(-1.8,0.,1.4));
#7383=CARTESIAN_POINT('',(-2.2,-4.89858719658941E-17,1.9));
#7384=CARTESIAN_POINT('',(-2.2,-4.89858719658941E-17,0.9));
#7385=CARTESIAN_POINT('Origin',(-1.8,0.,2.3));
#7386=CARTESIAN_POINT('',(-1.6,-0.346410161513776,2.1));
#7387=CARTESIAN_POINT('Origin',(-1.8,0.,2.3));
#7388=CARTESIAN_POINT('',(-1.6,-0.346410161513776,0.9));
#7389=CARTESIAN_POINT('',(-1.6,0.346410161513776,2.1));
#7390=CARTESIAN_POINT('',(-1.6,0.346410161513776,0.9));
#7391=CARTESIAN_POINT('Origin',(-1.8,0.,2.3));
#7392=CARTESIAN_POINT('Origin',(-1.8,0.,2.3));
#7393=CARTESIAN_POINT('Origin',(-1.6,0.,2.3));
#7394=CARTESIAN_POINT('',(-1.6,-4.89858719658941E-17,2.7));
#7395=CARTESIAN_POINT('Origin',(-1.6,0.,2.3));
#7396=CARTESIAN_POINT('Origin',(-1.6,0.,2.3));
#7397=CARTESIAN_POINT('Origin',(-3.1,0.,2.3));
#7398=CARTESIAN_POINT('',(-3.,-4.89858719658941E-17,2.7));
#7399=CARTESIAN_POINT('Origin',(-3.,0.,2.3));
#7400=CARTESIAN_POINT('',(-3.1,-4.89858719658941E-17,2.7));
#7401=CARTESIAN_POINT('Origin',(-4.6,0.,2.3));
#7402=CARTESIAN_POINT('',(-4.44755831889813,0.685,2.3));
#7403=CARTESIAN_POINT('',(-4.5,-8.38883057415937E-17,2.985));
#7404=CARTESIAN_POINT('Ctrl Pts',(-4.44755831889813,0.685,2.3));
#7405=CARTESIAN_POINT('Ctrl Pts',(-4.44755831889813,0.685,2.38615495576053));
#7406=CARTESIAN_POINT('Ctrl Pts',(-4.4503204226392,0.667754444280465,2.47795945171461));
#7407=CARTESIAN_POINT('Ctrl Pts',(-4.46025507446226,0.597806423657171,2.64668870614449));
#7408=CARTESIAN_POINT('Ctrl Pts',(-4.46727957365527,0.545111157186078,2.72362513303949));
#7409=CARTESIAN_POINT('Ctrl Pts',(-4.48043230270009,0.42362625704472,2.84511003318085));
#7410=CARTESIAN_POINT('Ctrl Pts',(-4.48742111878839,0.346689345476453,2.89780618135505));
#7411=CARTESIAN_POINT('Ctrl Pts',(-4.49727390705164,0.177958434129502,2.96775484339031));
#7412=CARTESIAN_POINT('Ctrl Pts',(-4.5,0.0861533615257772,2.985));
#7413=CARTESIAN_POINT('Ctrl Pts',(-4.5,1.11022302462516E-16,2.985));
#7414=CARTESIAN_POINT('',(-4.5,-3.58812256655041E-16,1.615));
#7415=CARTESIAN_POINT('Ctrl Pts',(-4.5,-1.66533453693773E-16,1.615));
#7416=CARTESIAN_POINT('Ctrl Pts',(-4.5,0.0861533615257768,1.615));
#7417=CARTESIAN_POINT('Ctrl Pts',(-4.49727390705164,0.177958434129502,1.63224515660969));
#7418=CARTESIAN_POINT('Ctrl Pts',(-4.48742111878839,0.346689345476453,1.70219381864495));
#7419=CARTESIAN_POINT('Ctrl Pts',(-4.48043230270009,0.42362625704472,1.75488996681915));
#7420=CARTESIAN_POINT('Ctrl Pts',(-4.46727957365527,0.545111157186078,1.87637486696051));
#7421=CARTESIAN_POINT('Ctrl Pts',(-4.46025507446226,0.597806423657171,1.95331129385551));
#7422=CARTESIAN_POINT('Ctrl Pts',(-4.4503204226392,0.667754444280465,2.12204054828539));
#7423=CARTESIAN_POINT('Ctrl Pts',(-4.44755831889813,0.685,2.21384504423947));
#7424=CARTESIAN_POINT('Ctrl Pts',(-4.44755831889813,0.685,2.3));
#7425=CARTESIAN_POINT('Ctrl Pts',(-4.5,1.11022302462516E-16,2.985));
#7426=CARTESIAN_POINT('Ctrl Pts',(-4.5,-0.0861533615257769,2.985));
#7427=CARTESIAN_POINT('Ctrl Pts',(-4.49727390705164,-0.177958434129502,
2.96775484339031));
#7428=CARTESIAN_POINT('Ctrl Pts',(-4.48742111878839,-0.346689345476453,
2.89780618135505));
#7429=CARTESIAN_POINT('Ctrl Pts',(-4.48043230270009,-0.42362625704472,2.84511003318085));
#7430=CARTESIAN_POINT('Ctrl Pts',(-4.46727957365527,-0.545111157186078,
2.72362513303949));
#7431=CARTESIAN_POINT('Ctrl Pts',(-4.46025507446226,-0.597806423657171,
2.64668870614449));
#7432=CARTESIAN_POINT('Ctrl Pts',(-4.4503204226392,-0.667754444280465,2.47795945171461));
#7433=CARTESIAN_POINT('Ctrl Pts',(-4.44755831889813,-0.685,2.38615495576053));
#7434=CARTESIAN_POINT('Ctrl Pts',(-4.44755831889813,-0.685,2.21384504423947));
#7435=CARTESIAN_POINT('Ctrl Pts',(-4.4503204226392,-0.667754444280465,2.12204054828539));
#7436=CARTESIAN_POINT('Ctrl Pts',(-4.46025507446226,-0.597806423657171,
1.95331129385551));
#7437=CARTESIAN_POINT('Ctrl Pts',(-4.46727957365527,-0.545111157186078,
1.87637486696051));
#7438=CARTESIAN_POINT('Ctrl Pts',(-4.48043230270009,-0.42362625704472,1.75488996681915));
#7439=CARTESIAN_POINT('Ctrl Pts',(-4.48742111878839,-0.346689345476453,
1.70219381864495));
#7440=CARTESIAN_POINT('Ctrl Pts',(-4.49727390705164,-0.177958434129502,
1.63224515660969));
#7441=CARTESIAN_POINT('Ctrl Pts',(-4.5,-0.0861533615257771,1.615));
#7442=CARTESIAN_POINT('Ctrl Pts',(-4.5,-1.38777878078145E-16,1.615));
#7443=CARTESIAN_POINT('',(-3.,-8.38883057415937E-17,2.985));
#7444=CARTESIAN_POINT('',(-4.6,-8.38883057415937E-17,2.985));
#7445=CARTESIAN_POINT('Origin',(-3.,0.,2.3));
#7446=CARTESIAN_POINT('Origin',(-3.,0.,2.3));
#7447=CARTESIAN_POINT('Origin',(0.,0.,0.76));
#7448=CARTESIAN_POINT('',(-0.89,-1.08993565124114E-16,0.76));
#7449=CARTESIAN_POINT('Origin',(0.,0.,0.76));
#7450=CARTESIAN_POINT('',(-0.89,-1.08993565124114E-16,1.04));
#7451=CARTESIAN_POINT('',(-0.89,-1.08993565124114E-16,0.76));
#7452=CARTESIAN_POINT('Origin',(0.,0.,1.04));
#7453=CARTESIAN_POINT('Origin',(0.,0.,1.04));
#7454=CARTESIAN_POINT('',(-0.6185,7.57444045272638E-17,1.04));
#7455=CARTESIAN_POINT('Origin',(0.,0.,1.04));
#7456=CARTESIAN_POINT('Origin',(0.,0.,0.76));
#7457=CARTESIAN_POINT('',(-0.6185,-7.57444045272638E-17,0.76));
#7458=CARTESIAN_POINT('Origin',(0.,0.,0.76));
#7459=CARTESIAN_POINT('Origin',(0.,0.,0.4));
#7460=CARTESIAN_POINT('',(-0.6185,-7.57444045272638E-17,0.5));
#7461=CARTESIAN_POINT('Origin',(0.,0.,0.5));
#7462=CARTESIAN_POINT('',(-0.6185,-7.57444045272638E-17,0.4));
#7463=CARTESIAN_POINT('Origin',(0.,0.,0.4));
#7464=CARTESIAN_POINT('',(-0.6185,-7.57444045272638E-17,1.5));
#7465=CARTESIAN_POINT('',(-0.6185,-7.57444045272638E-17,0.4));
#7466=CARTESIAN_POINT('Origin',(0.,0.,1.5));
#7467=CARTESIAN_POINT('Origin',(0.,0.,0.5));
#7468=CARTESIAN_POINT('',(-1.1,-1.34711147906209E-16,1.4));
#7469=CARTESIAN_POINT('Origin',(0.,0.,1.4));
#7470=CARTESIAN_POINT('',(-1.1,-1.34711147906209E-16,0.5));
#7471=CARTESIAN_POINT('',(-1.1,-1.34711147906209E-16,0.5));
#7472=CARTESIAN_POINT('Origin',(0.,0.,0.5));
#7473=CARTESIAN_POINT('Origin',(0.,0.,1.5));
#7474=CARTESIAN_POINT('',(-0.8,9.79717439317883E-17,1.5));
#7475=CARTESIAN_POINT('Origin',(0.,0.,1.5));
#7476=CARTESIAN_POINT('Origin',(0.,0.,0.5));
#7477=CARTESIAN_POINT('Origin',(0.,0.,2.3));
#7478=CARTESIAN_POINT('',(-0.6,-7.34788079488412E-17,2.4));
#7479=CARTESIAN_POINT('Origin',(0.,0.,2.4));
#7480=CARTESIAN_POINT('',(-0.6,7.34788079488412E-17,3.2));
#7481=CARTESIAN_POINT('',(-0.6,-7.34788079488412E-17,2.3));
#7482=CARTESIAN_POINT('Origin',(0.,0.,3.2));
#7483=CARTESIAN_POINT('Origin',(0.,0.,1.4));
#7484=CARTESIAN_POINT('',(-0.8,-9.79717439317883E-17,2.4));
#7485=CARTESIAN_POINT('',(-0.8,-9.79717439317883E-17,1.4));
#7486=CARTESIAN_POINT('Origin',(0.,0.,2.4));
#7487=CARTESIAN_POINT('Origin',(0.,0.,2.4));
#7488=CARTESIAN_POINT('Origin',(0.,0.,3.2));
#7489=CARTESIAN_POINT('',(-2.5,-3.06161699786838E-16,3.2));
#7490=CARTESIAN_POINT('Origin',(0.,0.,3.2));
#7491=CARTESIAN_POINT('',(-2.5,3.06161699786838E-16,5.));
#7492=CARTESIAN_POINT('',(-2.5,-3.06161699786838E-16,3.2));
#7493=CARTESIAN_POINT('Origin',(0.,0.,5.));
#7494=CARTESIAN_POINT('Origin',(0.,0.,3.2));
#7495=CARTESIAN_POINT('Origin',(0.,0.,0.9));
#7496=CARTESIAN_POINT('',(-3.31,-4.05358090517774E-16,1.));
#7497=CARTESIAN_POINT('Origin',(0.,0.,1.));
#7498=CARTESIAN_POINT('',(-3.31,-4.05358090517774E-16,0.9));
#7499=CARTESIAN_POINT('Origin',(0.,0.,1.4));
#7500=CARTESIAN_POINT('Origin',(0.,0.,1.));
#7501=CARTESIAN_POINT('',(-4.5,-5.51091059616309E-16,5.));
#7502=CARTESIAN_POINT('Origin',(0.,0.,5.));
#7503=CARTESIAN_POINT('',(-4.5,-5.51091059616309E-16,1.));
#7504=CARTESIAN_POINT('',(-4.5,-5.51091059616309E-16,1.));
#7505=CARTESIAN_POINT('',(-4.5,-5.51091059616309E-16,1.));
#7506=CARTESIAN_POINT('Origin',(0.,0.,1.));
#7507=CARTESIAN_POINT('Origin',(0.,0.,5.));
#7508=CARTESIAN_POINT('Origin',(0.,0.,1.));
#10218=UNCERTAINTY_MEASURE_WITH_UNIT(LENGTH_MEASURE(0.001),#10267,
'DISTANCE_ACCURACY_VALUE',
'Maximum model space distance between geometric entities at asserted c
onnectivities');
#10241=UNCERTAINTY_MEASURE_WITH_UNIT(LENGTH_MEASURE(0.001),#10267,
'DISTANCE_ACCURACY_VALUE',
'Maximum model space distance between geometric entities at asserted c
onnectivities');
#10243=(
GEOMETRIC_REPRESENTATION_CONTEXT(3)
GLOBAL_UNCERTAINTY_ASSIGNED_CONTEXT((#10218))
GLOBAL_UNIT_ASSIGNED_CONTEXT((#10267,#10269,#10270))
REPRESENTATION_CONTEXT('','3D')
);
#10266=(
GEOMETRIC_REPRESENTATION_CONTEXT(3)
GLOBAL_UNCERTAINTY_ASSIGNED_CONTEXT((#10241))
GLOBAL_UNIT_ASSIGNED_CONTEXT((#10267,#10269,#10270))
REPRESENTATION_CONTEXT('','3D')
);
#10267=(
LENGTH_UNIT()
NAMED_UNIT(*)
SI_UNIT(.CENTI.,.METRE.)
);
#10269=(
NAMED_UNIT(*)
PLANE_ANGLE_UNIT()
SI_UNIT($,.RADIAN.)
);
#10270=(
NAMED_UNIT(*)
SI_UNIT($,.STERADIAN.)
SOLID_ANGLE_UNIT()
);
#10272=SHAPE_DEFINITION_REPRESENTATION(#10296,#10355);
#10296=PRODUCT_DEFINITION_SHAPE('',$,#10380);
#10355=SHAPE_REPRESENTATION('',(#4971),#10243);
#10378=PRODUCT_DEFINITION_CONTEXT('part definition',#10452,'design');
#10380=PRODUCT_DEFINITION('Filter regulator body',
'Filter regulator body',#10404,#10378);
#10404=PRODUCT_DEFINITION_FORMATION('',$,#10455);
#10452=APPLICATION_CONTEXT(
'Core Data for Automotive Mechanical Design Process');
#10453=PRODUCT_CONTEXT('part definition',#10452,'mechanical');
#10455=PRODUCT('Filter regulator body','Filter regulator body',
'Filter regulator body',(#10453));
#10520=COLOUR_RGB('Dark Blue',0.08,0.2,0.34);
#10521=FILL_AREA_STYLE_COLOUR('',#10520);
#10522=FILL_AREA_STYLE('',(#10521));
#10523=SURFACE_STYLE_FILL_AREA(#10522);
#10524=SURFACE_SIDE_STYLE('',(#10523));
#10525=SURFACE_STYLE_USAGE(.BOTH.,#10524);
#10526=PRESENTATION_STYLE_ASSIGNMENT((#10525));
ENDSEC;
END-ISO-10303-21;
